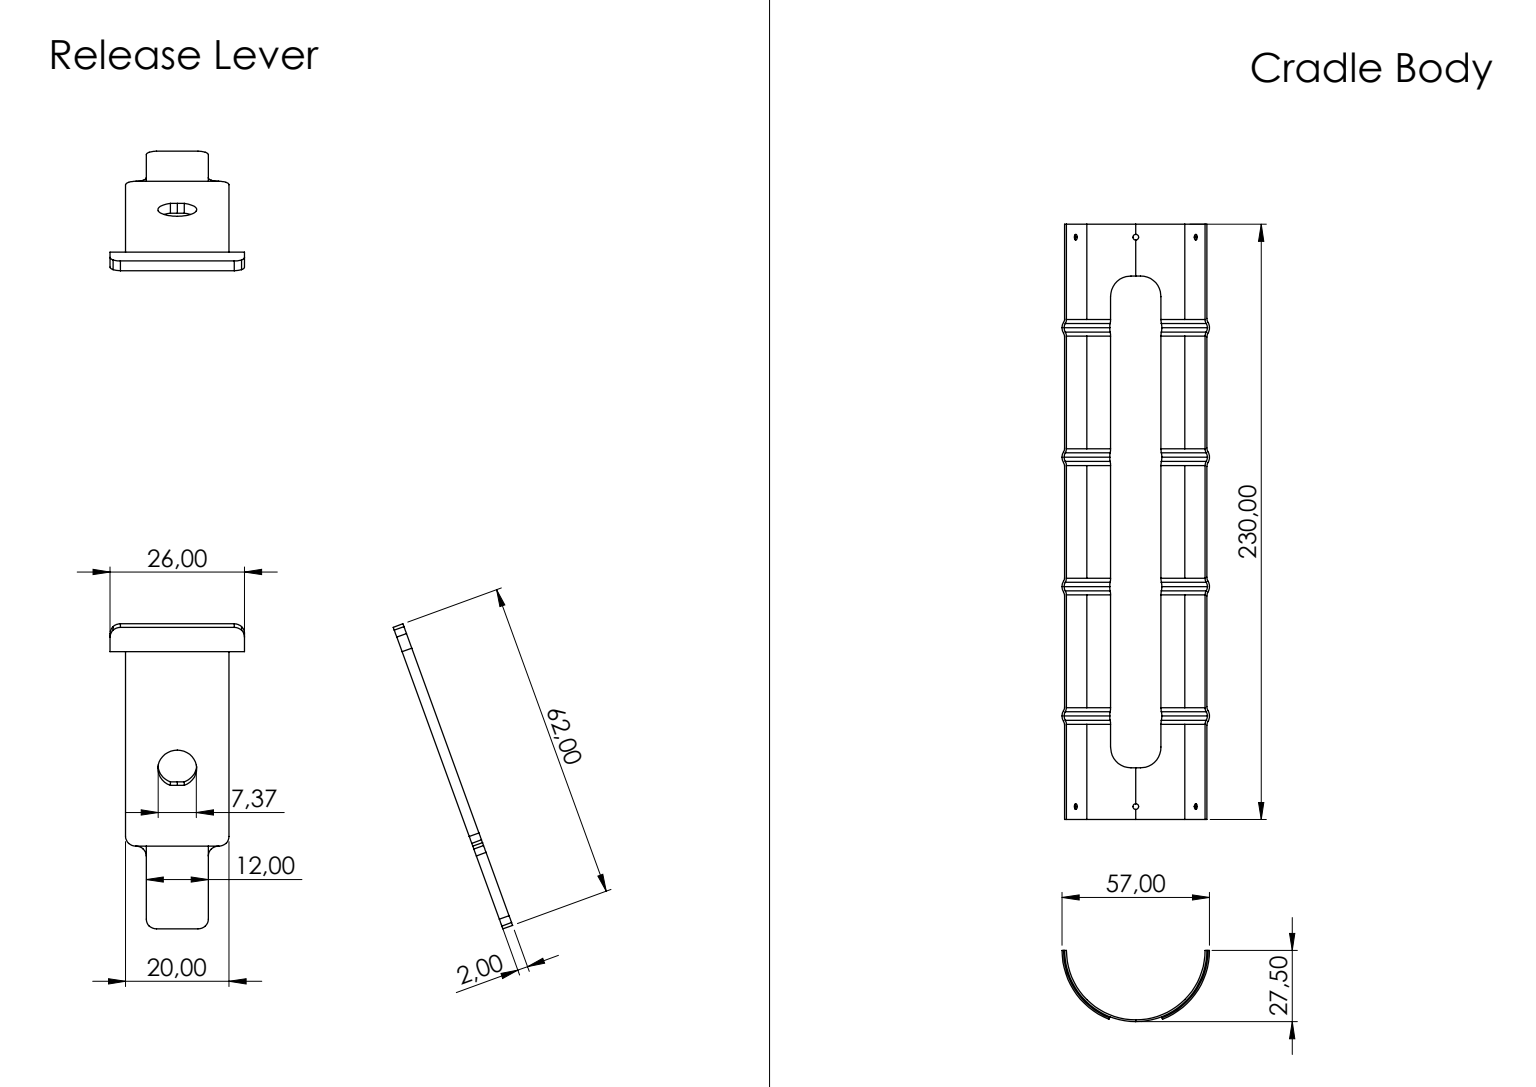
ISO-10303-21;
HEADER;
FILE_DESCRIPTION (('STEP AP214'),
    '1' );
FILE_NAME ('Release Lever.step',
    '2026-10-06T09:00:30',
    ( '' ),
    ( '' ),
    'SwSTEP 2.0',
    'SolidWorks 2020',
    '' );
FILE_SCHEMA (( 'AUTOMOTIVE_DESIGN' ));
ENDSEC;

DATA;
#27=EDGE_CURVE ( 'NONE', #20783, #1709, #15444, .T. ) ;
#39=CARTESIAN_POINT ( 'NONE',  ( 5.746322866173966482, -30.90925660337144265, -80.12837891589188644 ) ) ;
#44=CARTESIAN_POINT ( 'NONE',  ( 1.346291201779999946, -4.118494162357343669, -70.37733883405731206 ) ) ;
#60=CARTESIAN_POINT ( 'NONE',  ( -1.682270644565667439, 2.346032993262427091, -68.02444337080407877 ) ) ;
#66=DIRECTION ( 'NONE',  ( 0.000000000000000000, -0.3420201433259318913, 0.9396926207858126157 ) ) ;
#94=ORIENTED_EDGE ( 'NONE', *, *, #1377, .F. ) ;
#102=CARTESIAN_POINT ( 'NONE',  ( -10.00000000000000000, 21.72305290929948640, -60.97178489257708378 ) ) ;
#116=CARTESIAN_POINT ( 'NONE',  ( -6.000000000000000000, -30.08462078616447499, -79.82823602431849963 ) ) ;
#118=CARTESIAN_POINT ( 'NONE',  ( -8.261799387992772026, -15.86465192213916353, -74.65259062561661096 ) ) ;
#129=AXIS2_PLACEMENT_3D ( 'NONE', #21311, #28843, #21003 ) ;
#132=ORIENTED_EDGE ( 'NONE', *, *, #23382, .F. ) ;
#139=CARTESIAN_POINT ( 'NONE',  ( 0.000000000000000000, 5.495185456771864096, -69.00660115587162124 ) ) ;
#141=CYLINDRICAL_SURFACE ( 'NONE', #31028, 3.749999999999999556 ) ;
#143=CIRCLE ( 'NONE', #28760, 2.000000000000000000 ) ;
#148=CARTESIAN_POINT ( 'NONE',  ( 4.000000000000000000, -31.49740633216590524, -81.40662568294101220 ) ) ;
#151=CARTESIAN_POINT ( 'NONE',  ( 4.000000000000000000, -29.96004123392021157, -79.78289277550334191 ) ) ;
#168=ORIENTED_EDGE ( 'NONE', *, *, #10296, .F. ) ;
#201=DIRECTION ( 'NONE',  ( 0.000000000000000000, 0.3420201433259318913, -0.9396926207858126157 ) ) ;
#218=LINE ( 'NONE', #7132, #8498 ) ;
#267=DIRECTION ( 'NONE',  ( -1.000000000000000000, 0.000000000000000000, 0.000000000000000000 ) ) ;
#348=LINE ( 'NONE', #2999, #25253 ) ;
#359=VERTEX_POINT ( 'NONE', #2030 ) ;
#376=LINE ( 'NONE', #19562, #18555 ) ;
#394=ORIENTED_EDGE ( 'NONE', *, *, #19312, .F. ) ;
#425=DIRECTION ( 'NONE',  ( -1.000000000000000000, 0.000000000000000000, 0.000000000000000000 ) ) ;
#430=CARTESIAN_POINT ( 'NONE',  ( -6.000000000000000000, -29.96004123392021157, -79.78289277550334191 ) ) ;
#446=EDGE_CURVE ( 'NONE', #1677, #8641, #13828, .T. ) ;
#476=AXIS2_PLACEMENT_3D ( 'NONE', #10659, #13016, #25296 ) ;
#506=CARTESIAN_POINT ( 'NONE',  ( 9.229093439197374238, -15.48814874288954613, -74.51555467526300447 ) ) ;
#507=CARTESIAN_POINT ( 'NONE',  ( 5.601646981916513113, -31.11278470850464473, -80.20245708799704687 ) ) ;
#526=FILL_AREA_STYLE_COLOUR ( '', #18851 ) ;
#533=ORIENTED_EDGE ( 'NONE', *, *, #12374, .F. ) ;
#544=APPLICATION_CONTEXT ( 'automotive_design' ) ;
#572=( LENGTH_UNIT ( ) NAMED_UNIT ( * ) SI_UNIT ( .MILLI., .METRE. ) );
#634=ORIENTED_EDGE ( 'NONE', *, *, #28989, .F. ) ;
#639=PRODUCT_CONTEXT ( 'NONE', #19223, 'mechanical' ) ;
#645=CARTESIAN_POINT ( 'NONE',  ( -6.585786437629999490, -15.73107082825028336, -76.73232662853232000 ) ) ;
#653=CARTESIAN_POINT ( 'NONE',  ( 3.686970300939999667, -0.1862064327014488485, -68.94610314789109395 ) ) ;
#665=EDGE_LOOP ( 'NONE', ( #12496, #18069, #19743, #15909 ) ) ;
#670=CARTESIAN_POINT ( 'NONE',  ( 9.947945353310727157, -14.47719179179285476, -74.14759643693901126 ) ) ;
#703=DIRECTION ( 'NONE',  ( -1.000000000000000000, 0.000000000000000000, 0.000000000000000000 ) ) ;
#724=DIRECTION ( 'NONE',  ( 0.000000000000000000, -0.3420201433259318358, 0.9396926207858125046 ) ) ;
#759=AXIS2_PLACEMENT_3D ( 'NONE', #15036, #8234, #5426 ) ;
#767=B_SPLINE_CURVE_WITH_KNOTS ( 'NONE', 3,
 ( #13205, #8639, #22518, #965, #1269, #18235 ),
 .UNSPECIFIED., .F., .F.,
 ( 4, 2, 4 ),
 ( 0.000000000000000000, 0.5000000000000000000, 1.000000000000000000 ),
 .UNSPECIFIED. ) ;
#787=ADVANCED_FACE ( 'NONE', ( #14575 ), #4508, .F. ) ;
#816=CARTESIAN_POINT ( 'NONE',  ( -8.000000000000000000, -17.05999687705277879, -77.21601615383784178 ) ) ;
#826=ORIENTED_EDGE ( 'NONE', *, *, #17759, .F. ) ;
#877=DIRECTION ( 'NONE',  ( -0.000000000000000000, -0.9396926207858126157, -0.3420201433259318913 ) ) ;
#894=ORIENTED_EDGE ( 'NONE', *, *, #4532, .F. ) ;
#933=AXIS2_PLACEMENT_3D ( 'NONE', #27960, #6400, #18514 ) ;
#941=MANIFOLD_SOLID_BREP ( 'PartBody', #9536 ) ;
#949=CARTESIAN_POINT ( 'NONE',  ( 8.000000000050000892, -13.98526668056139144, -73.96855033896248699 ) ) ;
#965=CARTESIAN_POINT ( 'NONE',  ( -9.947945353463017781, -14.47719179108256782, -74.14759643668045896 ) ) ;
#1023=PRESENTATION_STYLE_ASSIGNMENT (( #20206 ) ) ;
#1039=FACE_OUTER_BOUND ( 'NONE', #21921, .T. ) ;
#1080=ORIENTED_EDGE ( 'NONE', *, *, #19351, .T. ) ;
#1104=CARTESIAN_POINT ( 'NONE',  ( -11.50000000000000000, 22.40709319595134730, -62.85117013414870257 ) ) ;
#1176=EDGE_CURVE ( 'NONE', #24619, #15474, #22131, .T. ) ;
#1181=DIRECTION ( 'NONE',  ( 0.9831920802501790124, -0.1715636151751586680, -0.06244404920691486172 ) ) ;
#1199=CARTESIAN_POINT ( 'NONE',  ( 10.00000000000000000, 21.72305290929948640, -60.97178489257708378 ) ) ;
#1210=AXIS2_PLACEMENT_3D ( 'NONE', #8253, #3381, #5296 ) ;
#1247=ORIENTED_EDGE ( 'NONE', *, *, #9957, .T. ) ;
#1248=AXIS2_PLACEMENT_3D ( 'NONE', #26035, #21308, #6364 ) ;
#1269=CARTESIAN_POINT ( 'NONE',  ( -10.00000000005000445, -14.23127763322419703, -74.05809100303530101 ) ) ;
#1274=ORIENTED_EDGE ( 'NONE', *, *, #21907, .T. ) ;
#1281=CARTESIAN_POINT ( 'NONE',  ( 6.000000000000000000, -17.74403716370463968, -75.33663091226621589 ) ) ;
#1284=SURFACE_STYLE_USAGE ( .BOTH. , #7880 ) ;
#1293=CARTESIAN_POINT ( 'NONE',  ( -8.000000000000000000, -17.74403716370463968, -75.33663091226621589 ) ) ;
#1321=CARTESIAN_POINT ( 'NONE',  ( -3.686970300939999667, -0.1862064327014488485, -68.94610314789107974 ) ) ;
#1336=CARTESIAN_POINT ( 'NONE',  ( -4.000000000000000000, -29.27600094726834712, -81.66227801707495360 ) ) ;
#1347=VERTEX_POINT ( 'NONE', #9746 ) ;
#1370=B_SPLINE_CURVE_WITH_KNOTS ( 'NONE', 3,
 ( #653, #3728, #17314, #26919, #19984, #11129, #26759, #24707, #25292, #6250 ),
 .UNSPECIFIED., .F., .F.,
 ( 4, 2, 2, 2, 4 ),
 ( 0.000000000000000000, 0.2500000000000000000, 0.5000000000000000000, 0.7500000000000000000, 1.000000000000000000 ),
 .UNSPECIFIED. ) ;
#1377=EDGE_CURVE ( 'NONE', #21922, #24619, #143, .T. ) ;
#1378=CARTESIAN_POINT ( 'NONE',  ( -8.000000000000000000, -15.86465192213301556, -74.65259062561435144 ) ) ;
#1392=LINE ( 'NONE', #16015, #6709 ) ;
#1399=AXIS2_PLACEMENT_3D ( 'NONE', #949, #20134, #22648 ) ;
#1472=DIRECTION ( 'NONE',  ( 0.000000000000000000, 0.3420201433259318913, -0.9396926207858126157 ) ) ;
#1496=AXIS2_PLACEMENT_3D ( 'NONE', #1293, #13078, #29613 ) ;
#1517=CARTESIAN_POINT ( 'NONE',  ( 1.070547230664766758, 2.553693132251782405, -67.94886126136832161 ) ) ;
#1528=EDGE_CURVE ( 'NONE', #24268, #24784, #17639, .T. ) ;
#1533=CARTESIAN_POINT ( 'NONE',  ( 8.000000000000000000, -15.86465192213301556, -74.65259062561435144 ) ) ;
#1567=EDGE_CURVE ( 'NONE', #13375, #14059, #30931, .T. ) ;
#1573=CARTESIAN_POINT ( 'NONE',  ( 11.00000000000000000, 26.42151601322854759, -59.26168417594741555 ) ) ;
#1597=EDGE_LOOP ( 'NONE', ( #9088, #27743, #23180, #6425 ) ) ;
#1608=VECTOR ( 'NONE', #14619, 1000.000000000000114 ) ;
#1661=CARTESIAN_POINT ( 'NONE',  ( 8.000000000050000892, -13.98526668056139144, -73.96855033896248699 ) ) ;
#1677=VERTEX_POINT ( 'NONE', #1281 ) ;
#1694=DIRECTION ( 'NONE',  ( 0.000000000000000000, 0.3420201433259318358, -0.9396926207858125046 ) ) ;
#1702=ORIENTED_EDGE ( 'NONE', *, *, #26033, .F. ) ;
#1709=VERTEX_POINT ( 'NONE', #28014 ) ;
#1710=CIRCLE ( 'NONE', #5716, 2.000000000000000000 ) ;
#1758=AXIS2_PLACEMENT_3D ( 'NONE', #6175, #1472, #20659 ) ;
#1791=LINE ( 'NONE', #25394, #9769 ) ;
#1855=LINE ( 'NONE', #16324, #16326 ) ;
#1890=LINE ( 'NONE', #6760, #17257 ) ;
#1892=EDGE_CURVE ( 'NONE', #3795, #15436, #7619, .T. ) ;
#1894=CARTESIAN_POINT ( 'NONE',  ( -3.629744515141296368, -1.804033921010813835, -69.53494419781382874 ) ) ;
#1895=ORIENTED_EDGE ( 'NONE', *, *, #2972, .T. ) ;
#1912=AXIS2_PLACEMENT_3D ( 'NONE', #21616, #66, #9646 ) ;
#1918=PLANE ( 'NONE',  #23555 ) ;
#1930=CARTESIAN_POINT ( 'NONE',  ( -6.000000000000000000, -23.85203919881242385, -77.55976184388477179 ) ) ;
#1939=ORIENTED_EDGE ( 'NONE', *, *, #28404, .T. ) ;
#1980=CARTESIAN_POINT ( 'NONE',  ( 0.000000000000000000, 27.10555629988041204, -61.14106941751904856 ) ) ;
#1986=ADVANCED_FACE ( 'NONE', ( #30114, #6190 ), #13906, .F. ) ;
#1999=LINE ( 'NONE', #29299, #4426 ) ;
#2027=ORIENTED_EDGE ( 'NONE', *, *, #20844, .F. ) ;
#2030=CARTESIAN_POINT ( 'NONE',  ( -10.00000000000000000, -13.98526668056139144, -73.96855033896248699 ) ) ;
#2106=DIRECTION ( 'NONE',  ( 0.000000000000000000, -0.3420201433259318913, 0.9396926207858126157 ) ) ;
#2111=VERTEX_POINT ( 'NONE', #9019 ) ;
#2145=ORIENTED_EDGE ( 'NONE', *, *, #29497, .T. ) ;
#2148=DIRECTION ( 'NONE',  ( 0.000000000000000000, -0.3420201433259318358, 0.9396926207858125046 ) ) ;
#2167=CARTESIAN_POINT ( 'NONE',  ( 12.41421356240000051, 26.55509710711128335, -61.34142017886538412 ) ) ;
#2201=LINE ( 'NONE', #4866, #16643 ) ;
#2209=CARTESIAN_POINT ( 'NONE',  ( -1.750888960315145848, -3.972249423281244862, -70.32411010211554014 ) ) ;
#2211=CIRCLE ( 'NONE', #10247, 3.750000000000000000 ) ;
#2254=DIRECTION ( 'NONE',  ( 0.000000000000000000, 0.9396926207858125046, 0.3420201433259318358 ) ) ;
#2256=EDGE_LOOP ( 'NONE', ( #634, #29786, #11374, #18353 ) ) ;
#2258=VERTEX_POINT ( 'NONE', #26478 ) ;
#2291=FACE_OUTER_BOUND ( 'NONE', #5378, .T. ) ;
#2296=( GEOMETRIC_REPRESENTATION_CONTEXT ( 3 ) GLOBAL_UNCERTAINTY_ASSIGNED_CONTEXT ( ( #10001 ) ) GLOBAL_UNIT_ASSIGNED_CONTEXT ( ( #15439, #3164, #8338 ) ) REPRESENTATION_CONTEXT ( 'NONE', 'WORKASPACE' ) );
#2356=LINE ( 'NONE', #16655, #3079 ) ;
#2365=CARTESIAN_POINT ( 'NONE',  ( 5.999999999999997335, -17.49802621104079137, -75.24709024819303238 ) ) ;
#2368=ORIENTED_EDGE ( 'NONE', *, *, #11363, .T. ) ;
#2392=CARTESIAN_POINT ( 'NONE',  ( 8.261799387612766665, -15.86465192213917064, -74.65259062561659675 ) ) ;
#2433=DIRECTION ( 'NONE',  ( -1.000000000000000000, 0.000000000000000000, 0.000000000000000000 ) ) ;
#2440=DIRECTION ( 'NONE',  ( 0.000000000000000000, 0.3420201433259318913, -0.9396926207858126157 ) ) ;
#2442=VECTOR ( 'NONE', #2526, 1000.000000000000114 ) ;
#2468=CARTESIAN_POINT ( 'NONE',  ( -13.00000000000000000, 23.81663212713006672, -62.33813991915980779 ) ) ;
#2526=DIRECTION ( 'NONE',  ( 0.000000000000000000, 0.3420201433259318358, -0.9396926207858125046 ) ) ;
#2539=DIRECTION ( 'NONE',  ( 0.000000000000000000, -0.9396926207858125046, -0.3420201433259318358 ) ) ;
#2540=VECTOR ( 'NONE', #17749, 1000.000000000000114 ) ;
#2569=DIRECTION ( 'NONE',  ( 0.000000000000000000, 0.3420201433259318913, -0.9396926207858126157 ) ) ;
#2573=AXIS2_PLACEMENT_3D ( 'NONE', #24001, #2440, #18795 ) ;
#2616=CARTESIAN_POINT ( 'NONE',  ( 1.243449787579999883E-14, -31.15538618883996946, -82.34631830372681804 ) ) ;
#2627=CARTESIAN_POINT ( 'NONE',  ( 0.000000000000000000, 0.000000000000000000, 0.000000000000000000 ) ) ;
#2633=ORIENTED_EDGE ( 'NONE', *, *, #7472, .F. ) ;
#2672=VERTEX_POINT ( 'NONE', #14752 ) ;
#2691=CARTESIAN_POINT ( 'NONE',  ( 12.74757277707238856, 25.48862485010116075, -59.60122879113606587 ) ) ;
#2695=EDGE_CURVE ( 'NONE', #22118, #18765, #4850, .T. ) ;
#2708=CARTESIAN_POINT ( 'NONE',  ( 9.747572776401462136, -14.93176076027399901, -74.31304601088737627 ) ) ;
#2762=CARTESIAN_POINT ( 'NONE',  ( -11.00000000000000000, 25.22617105830878614, -61.82510970417090590 ) ) ;
#2772=CARTESIAN_POINT ( 'NONE',  ( -0.6731456008920000400, -3.434453875705480108, -72.25672407562892374 ) ) ;
#2813=CYLINDRICAL_SURFACE ( 'NONE', #24284, 2.000000000000003553 ) ;
#2814=LINE ( 'NONE', #22167, #18267 ) ;
#2817=ADVANCED_FACE ( 'NONE', ( #24932 ), #22423, .F. ) ;
#2827=ORIENTED_EDGE ( 'NONE', *, *, #2972, .F. ) ;
#2869=ORIENTED_EDGE ( 'NONE', *, *, #5232, .T. ) ;
#2891=LINE ( 'NONE', #17205, #10294 ) ;
#2917=CARTESIAN_POINT ( 'NONE',  ( -11.50000000000000000, 22.40709319595134730, -62.85117013414870257 ) ) ;
#2920=DIRECTION ( 'NONE',  ( 1.000000000000000000, -0.000000000000000000, 0.000000000000000000 ) ) ;
#2942=VECTOR ( 'NONE', #8951, 1000.000000000000114 ) ;
#2972=EDGE_CURVE ( 'NONE', #28085, #1347, #19245, .T. ) ;
#2975=EDGE_LOOP ( 'NONE', ( #13463, #826, #26860, #5305, #15473, #13542, #20696, #23812, #24583, #29901 ) ) ;
#2999=CARTESIAN_POINT ( 'NONE',  ( -13.00000000000000000, 22.06507305262541863, -61.91147751336289673 ) ) ;
#3020=EDGE_CURVE ( 'NONE', #31086, #17565, #15659, .T. ) ;
#3067=FACE_OUTER_BOUND ( 'NONE', #13010, .T. ) ;
#3075=EDGE_CURVE ( 'NONE', #359, #15474, #7131, .T. ) ;
#3079=VECTOR ( 'NONE', #21701, 1000.000000000000000 ) ;
#3103=AXIS2_PLACEMENT_3D ( 'NONE', #24128, #2106, #14381 ) ;
#3121=VERTEX_POINT ( 'NONE', #9644 ) ;
#3124=ORIENTED_EDGE ( 'NONE', *, *, #10955, .T. ) ;
#3156=CARTESIAN_POINT ( 'NONE',  ( -5.226724280842381276, -31.46509748598739975, -80.33068845215250064 ) ) ;
#3162=ORIENTED_EDGE ( 'NONE', *, *, #7689, .F. ) ;
#3164=( NAMED_UNIT ( * ) PLANE_ANGLE_UNIT ( ) SI_UNIT ( $, .RADIAN. ) );
#3201=EDGE_CURVE ( 'NONE', #24684, #1347, #376, .T. ) ;
#3202=ORIENTED_EDGE ( 'NONE', *, *, #23759, .F. ) ;
#3277=DIRECTION ( 'NONE',  ( 0.000000000000000000, -0.3420201433259318913, 0.9396926207858126157 ) ) ;
#3280=ORIENTED_EDGE ( 'NONE', *, *, #21019, .F. ) ;
#3293=LINE ( 'NONE', #24402, #27778 ) ;
#3364=DIRECTION ( 'NONE',  ( 0.000000000000000000, -0.9396926207858125046, -0.3420201433259318358 ) ) ;
#3381=DIRECTION ( 'NONE',  ( 0.000000000000000000, 0.3420201433259318913, -0.9396926207858126157 ) ) ;
#3396=AXIS2_PLACEMENT_3D ( 'NONE', #10919, #6031, #8542 ) ;
#3414=DIRECTION ( 'NONE',  ( 0.000000000000000000, 0.3420201433259318913, -0.9396926207858126157 ) ) ;
#3449=DIRECTION ( 'NONE',  ( 0.000000000000000000, 0.3420201433259318913, -0.9396926207858126157 ) ) ;
#3456=CARTESIAN_POINT ( 'NONE',  ( 9.414213562409999625, -15.31419272936388687, -74.45223986426802298 ) ) ;
#3462=CARTESIAN_POINT ( 'NONE',  ( -4.000000000000000000, -31.83942647549183746, -80.46693306215520636 ) ) ;
#3463=ORIENTED_EDGE ( 'NONE', *, *, #18343, .T. ) ;
#3464=CARTESIAN_POINT ( 'NONE',  ( -11.00000000000000000, 27.10555629988041204, -61.14106941751904856 ) ) ;
#3466=ORIENTED_EDGE ( 'NONE', *, *, #9897, .T. ) ;
#3472=ORIENTED_EDGE ( 'NONE', *, *, #15387, .T. ) ;
#3481=EDGE_CURVE ( 'NONE', #2258, #24119, #10233, .T. ) ;
#3495=B_SPLINE_CURVE_WITH_KNOTS ( 'NONE', 3,
 ( #19220, #21591, #2691, #7107, #26304, #28969 ),
 .UNSPECIFIED., .F., .F.,
 ( 4, 2, 4 ),
 ( 0.000000000000000000, 0.5000000000000000000, 1.000000000000000000 ),
 .UNSPECIFIED. ) ;
#3521=ORIENTED_EDGE ( 'NONE', *, *, #29385, .F. ) ;
#3570=DIRECTION ( 'NONE',  ( 0.7071067811865467956, 0.6644630243886068266, 0.2418447626481644297 ) ) ;
#3628=VECTOR ( 'NONE', #19062, 1000.000000000000114 ) ;
#3630=CARTESIAN_POINT ( 'NONE',  ( -3.015466128627334985, 1.304460199876133819, -68.40354486441854931 ) ) ;
#3636=CARTESIAN_POINT ( 'NONE',  ( -12.41421356240000051, 25.87105682045942245, -59.46203493729375822 ) ) ;
#3649=CARTESIAN_POINT ( 'NONE',  ( 4.440892098500000496E-16, -0.1455297029551360921, -71.05965357398815740 ) ) ;
#3674=CARTESIAN_POINT ( 'NONE',  ( 6.000000000000000000, -23.16799891216055940, -79.43914708545641190 ) ) ;
#3689=FACE_OUTER_BOUND ( 'NONE', #23976, .T. ) ;
#3706=DIRECTION ( 'NONE',  ( -1.000000000000000000, 0.000000000000000000, 0.000000000000000000 ) ) ;
#3721=AXIS2_PLACEMENT_3D ( 'NONE', #2917, #877, #425 ) ;
#3726=LINE ( 'NONE', #30323, #10479 ) ;
#3728=CARTESIAN_POINT ( 'NONE',  ( 3.766879923516746942, -0.5905747970024824989, -69.09328119617570962 ) ) ;
#3744=AXIS2_PLACEMENT_3D ( 'NONE', #31113, #5131, #14744 ) ;
#3783=VECTOR ( 'NONE', #2539, 1000.000000000000114 ) ;
#3795=VERTEX_POINT ( 'NONE', #19012 ) ;
#3796=( NAMED_UNIT ( * ) PLANE_ANGLE_UNIT ( ) SI_UNIT ( $, .RADIAN. ) );
#3810=EDGE_CURVE ( 'NONE', #359, #7467, #16800, .T. ) ;
#3866=CARTESIAN_POINT ( 'NONE',  ( 3.454291557259786316, 0.6014336072404916633, -68.65942561803572630 ) ) ;
#3913=VECTOR ( 'NONE', #4734, 1000.000000000000114 ) ;
#3924=CARTESIAN_POINT ( 'NONE',  ( 8.000000000000000000, -15.86465192213301556, -74.65259062561435144 ) ) ;
#3961=CARTESIAN_POINT ( 'NONE',  ( -12.22909343913021551, 26.04501283399531530, -59.39872012629501086 ) ) ;
#4004=VECTOR ( 'NONE', #18311, 1000.000000000000000 ) ;
#4017=ORIENTED_EDGE ( 'NONE', *, *, #7464, .F. ) ;
#4024=CARTESIAN_POINT ( 'NONE',  ( 0.8593139071816520147, 2.606839092805549818, -67.92951771365525815 ) ) ;
#4032=ORIENTED_EDGE ( 'NONE', *, *, #27, .T. ) ;
#4062=ORIENTED_EDGE ( 'NONE', *, *, #14447, .F. ) ;
#4102=EDGE_LOOP ( 'NONE', ( #533, #28019, #19197, #15165, #11526, #3521, #18884, #25233, #20427, #3466 ) ) ;
#4198=CIRCLE ( 'NONE', #26331, 3.750000000000000000 ) ;
#4356=EDGE_LOOP ( 'NONE', ( #12880, #9635, #28055, #16249 ) ) ;
#4360=CARTESIAN_POINT ( 'NONE',  ( -1.346291201779999946, -4.118494162357343669, -70.37733883405731206 ) ) ;
#4383=LINE ( 'NONE', #11156, #20990 ) ;
#4418=ORIENTED_EDGE ( 'NONE', *, *, #30801, .F. ) ;
#4426=VECTOR ( 'NONE', #26640, 1000.000000000000114 ) ;
#4440=DIRECTION ( 'NONE',  ( 0.000000000000000000, 0.3420201433259318358, -0.9396926207858125046 ) ) ;
#4503=AXIS2_PLACEMENT_3D ( 'NONE', #17531, #27139, #21653 ) ;
#4508=PLANE ( 'NONE',  #25624 ) ;
#4532=EDGE_CURVE ( 'NONE', #9238, #25602, #14330, .T. ) ;
#4538=DIRECTION ( 'NONE',  ( -1.000000000000000000, 0.000000000000000000, 0.000000000000000000 ) ) ;
#4574=LINE ( 'NONE', #11966, #3913 ) ;
#4587=EDGE_CURVE ( 'NONE', #8607, #4930, #20356, .T. ) ;
#4687=EDGE_LOOP ( 'NONE', ( #26398, #94, #9751, #13440 ) ) ;
#4709=ADVANCED_FACE ( 'NONE', ( #11706 ), #28225, .T. ) ;
#4713=VECTOR ( 'NONE', #19034, 1000.000000000000114 ) ;
#4734=DIRECTION ( 'NONE',  ( 0.000000000000000000, 0.3420201433259318358, -0.9396926207858125046 ) ) ;
#4753=CARTESIAN_POINT ( 'NONE',  ( 9.007237960087341122, -15.62744792347586476, -74.56625543065413808 ) ) ;
#4766=CARTESIAN_POINT ( 'NONE',  ( -11.00000000000000000, 25.22617105830878614, -61.82510970417090590 ) ) ;
#4836=ADVANCED_FACE ( 'NONE', ( #29152 ), #14226, .F. ) ;
#4848=B_SPLINE_CURVE_WITH_KNOTS ( 'NONE', 3,
 ( #9368, #29150, #10122, #7597, #11739, #17190 ),
 .UNSPECIFIED., .F., .F.,
 ( 4, 2, 4 ),
 ( 0.000000000000000000, 0.5000000000000000000, 1.000000000000000000 ),
 .UNSPECIFIED. ) ;
#4850=LINE ( 'NONE', #10033, #10148 ) ;
#4853=DIRECTION ( 'NONE',  ( 0.000000000000000000, 0.3420201433259318913, -0.9396926207858126157 ) ) ;
#4866=CARTESIAN_POINT ( 'NONE',  ( -6.339027081030000540E-10, -3.776474019031412777, -71.31703145484311790 ) ) ;
#4870=CARTESIAN_POINT ( 'NONE',  ( 13.00000000000000000, 22.40709319595134730, -62.85117013414870257 ) ) ;
#4884=CARTESIAN_POINT ( 'NONE',  ( 6.000000000000000000, -17.74403716370463968, -75.33663091226621589 ) ) ;
#4886=ORIENTED_EDGE ( 'NONE', *, *, #14233, .F. ) ;
#4930=VERTEX_POINT ( 'NONE', #6005 ) ;
#4972=PLANE ( 'NONE',  #3721 ) ;
#4976=CARTESIAN_POINT ( 'NONE',  ( -5.936576268373215726, -30.44659052782209585, -79.95998223598701315 ) ) ;
#4990=FACE_OUTER_BOUND ( 'NONE', #14209, .T. ) ;
#5015=DIRECTION ( 'NONE',  ( -1.000000000000000000, 0.000000000000000000, 0.000000000000000000 ) ) ;
#5018=DIRECTION ( 'NONE',  ( 0.000000000000000000, 0.3420201433259318913, -0.9396926207858126157 ) ) ;
#5064=ORIENTED_EDGE ( 'NONE', *, *, #15160, .F. ) ;
#5131=DIRECTION ( 'NONE',  ( 0.000000000000000000, 0.3420201433259318913, -0.9396926207858126157 ) ) ;
#5192=ADVANCED_FACE ( 'NONE', ( #30409 ), #25690, .T. ) ;
#5200=LINE ( 'NONE', #30611, #10649 ) ;
#5232=EDGE_CURVE ( 'NONE', #2258, #2672, #26150, .T. ) ;
#5276=FILL_AREA_STYLE_COLOUR ( '', #6386 ) ;
#5288=LINE ( 'NONE', #2772, #10747 ) ;
#5295=STYLED_ITEM ( 'NONE', ( #18094 ), #9916 ) ;
#5296=DIRECTION ( 'NONE',  ( 0.000000000000000000, 0.9396926207858125046, 0.3420201433259318358 ) ) ;
#5305=ORIENTED_EDGE ( 'NONE', *, *, #25713, .T. ) ;
#5308=PRODUCT_DEFINITION_FORMATION_WITH_SPECIFIED_SOURCE ( 'ANY', '', #28241, .NOT_KNOWN. ) ;
#5345=CARTESIAN_POINT ( 'NONE',  ( -10.00000000000000000, 4.552933401020911042, -69.34955285734142194 ) ) ;
#5353=EDGE_LOOP ( 'NONE', ( #14979, #20824, #16001, #18891 ) ) ;
#5356=CARTESIAN_POINT ( 'NONE',  ( -7.867425209648341244, -15.86465192213301911, -74.65259062561435144 ) ) ;
#5368=VECTOR ( 'NONE', #12353, 1000.000000000000114 ) ;
#5377=EDGE_CURVE ( 'NONE', #9001, #24684, #1370, .T. ) ;
#5378=EDGE_LOOP ( 'NONE', ( #11345, #18822, #7457, #14477 ) ) ;
#5387=EDGE_CURVE ( 'NONE', #16796, #5989, #6660, .T. ) ;
#5426=DIRECTION ( 'NONE',  ( -1.000000000000000000, 0.000000000000000000, 0.000000000000000000 ) ) ;
#5451=VECTOR ( 'NONE', #24263, 1000.000000000000114 ) ;
#5532=CARTESIAN_POINT ( 'NONE',  ( -3.607824829760114760, 0.2143012804528021953, -68.80033026170877974 ) ) ;
#5571=AXIS2_PLACEMENT_3D ( 'NONE', #9859, #7495, #17089 ) ;
#5573=CYLINDRICAL_SURFACE ( 'NONE', #15534, 2.000000000000002665 ) ;
#5589=CARTESIAN_POINT ( 'NONE',  ( -9.229093440751908517, -15.48814874182538226, -74.51555467487568762 ) ) ;
#5654=ADVANCED_FACE ( 'NONE', ( #3689 ), #17994, .F. ) ;
#5705=ORIENTED_EDGE ( 'NONE', *, *, #1176, .F. ) ;
#5716=AXIS2_PLACEMENT_3D ( 'NONE', #816, #10406, #14977 ) ;
#5731=CARTESIAN_POINT ( 'NONE',  ( 6.000000000000000000, -16.12030425626696939, -76.87399601051191667 ) ) ;
#5740=VECTOR ( 'NONE', #13256, 1000.000000000000000 ) ;
#5747=ORIENTED_EDGE ( 'NONE', *, *, #19483, .T. ) ;
#5762=ORIENTED_EDGE ( 'NONE', *, *, #16574, .T. ) ;
#5788=CARTESIAN_POINT ( 'NONE',  ( 13.00000000000000000, 23.81663212713006672, -62.33813991915980779 ) ) ;
#5886=FACE_OUTER_BOUND ( 'NONE', #2256, .T. ) ;
#5900=AXIS2_PLACEMENT_3D ( 'NONE', #14288, #24651, #14748 ) ;
#5929=FACE_OUTER_BOUND ( 'NONE', #24195, .T. ) ;
#5943=AXIS2_PLACEMENT_3D ( 'NONE', #15885, #13838, #6747 ) ;
#5989=VERTEX_POINT ( 'NONE', #22399 ) ;
#6005=CARTESIAN_POINT ( 'NONE',  ( -5.414213562369999622, -30.60492699607083722, -82.14596754238048959 ) ) ;
#6007=DIRECTION ( 'NONE',  ( 0.000000000000000000, 0.3420201433259318358, -0.9396926207858125046 ) ) ;
#6028=DIRECTION ( 'NONE',  ( 0.000000000000000000, 0.3420201433259318913, -0.9396926207858126157 ) ) ;
#6031=DIRECTION ( 'NONE',  ( 0.000000000000000000, -0.3420201433259318913, 0.9396926207858126157 ) ) ;
#6035=DIRECTION ( 'NONE',  ( 0.000000000000000000, -0.9396926207858125046, -0.3420201433259318358 ) ) ;
#6108=VECTOR ( 'NONE', #9491, 1000.000000000000114 ) ;
#6118=CARTESIAN_POINT ( 'NONE',  ( 12.41421356240000051, 25.87105682045942245, -59.46203493729375822 ) ) ;
#6131=CARTESIAN_POINT ( 'NONE',  ( -11.00000000000000000, 27.10555629988041204, -61.14106941751904856 ) ) ;
#6133=ORIENTED_EDGE ( 'NONE', *, *, #1528, .T. ) ;
#6175=CARTESIAN_POINT ( 'NONE',  ( 0.000000000000000000, 4.811145170119999648, -67.12721591429999535 ) ) ;
#6190=FACE_OUTER_BOUND ( 'NONE', #19033, .T. ) ;
#6211=DIRECTION ( 'NONE',  ( 0.000000000000000000, 0.3420201433259318913, -0.9396926207858126157 ) ) ;
#6216=VECTOR ( 'NONE', #9116, 1000.000000000000114 ) ;
#6250=CARTESIAN_POINT ( 'NONE',  ( 1.346291201779999946, -4.118494162357343669, -70.37733883405731206 ) ) ;
#6273=ORIENTED_EDGE ( 'NONE', *, *, #12374, .T. ) ;
#6302=CARTESIAN_POINT ( 'NONE',  ( -1.346291201779999946, -4.118494162357343669, -70.37733883405731206 ) ) ;
#6327=LINE ( 'NONE', #20645, #14528 ) ;
#6337=CARTESIAN_POINT ( 'NONE',  ( 2.664535259099999805E-15, 2.694277338339796213, -67.89769279494430521 ) ) ;
#6364=DIRECTION ( 'NONE',  ( 0.000000000000000000, 0.9396926207858125046, 0.3420201433259318358 ) ) ;
#6386=COLOUR_RGB ( '', 0.66274510, 0.83137255, 0.94901961) ;
#6400=DIRECTION ( 'NONE',  ( 0.000000000000000000, 0.3420201433259318913, -0.9396926207858126157 ) ) ;
#6425=ORIENTED_EDGE ( 'NONE', *, *, #29890, .T. ) ;
#6428=ORIENTED_EDGE ( 'NONE', *, *, #23291, .T. ) ;
#6452=B_SPLINE_CURVE_WITH_KNOTS ( 'NONE', 3,
 ( #22055, #506, #4753, #22199, #2392, #10090 ),
 .UNSPECIFIED., .F., .F.,
 ( 4, 2, 4 ),
 ( 0.000000000000000000, 0.5000000000000000000, 1.000000000000000000 ),
 .UNSPECIFIED. ) ;
#6473=VERTEX_POINT ( 'NONE', #16713 ) ;
#6484=CARTESIAN_POINT ( 'NONE',  ( 0.000000000000000000, 4.811145170119999648, -67.12721591429999535 ) ) ;
#6529=CYLINDRICAL_SURFACE ( 'NONE', #12771, 2.000000000000000000 ) ;
#6563=EDGE_CURVE ( 'NONE', #22118, #27093, #29447, .T. ) ;
#6585=AXIS2_PLACEMENT_3D ( 'NONE', #9296, #7252, #11663 ) ;
#6592=PLANE ( 'NONE',  #5943 ) ;
#6606=CARTESIAN_POINT ( 'NONE',  ( 5.228182028002445136, -31.46370949612416723, -80.33018326515686169 ) ) ;
#6650=CIRCLE ( 'NONE', #15180, 2.000000000000000000 ) ;
#6659=CARTESIAN_POINT ( 'NONE',  ( 6.585786437629999490, -16.41511111490214603, -74.85294138696069410 ) ) ;
#6660=B_SPLINE_CURVE_WITH_KNOTS ( 'NONE', 3,
 ( #1378, #5356, #27068, #14961, #13327, #10088, #27639, #12588 ),
 .UNSPECIFIED., .F., .F.,
 ( 4, 2, 2, 4 ),
 ( 0.000000000000000000, 0.2499999999999985567, 0.4999999999999971134, 1.000000000000000000 ),
 .UNSPECIFIED. ) ;
#6709=VECTOR ( 'NONE', #30806, 1000.000000000000114 ) ;
#6741=CARTESIAN_POINT ( 'NONE',  ( -10.00000000000000000, 3.868893114322062843, -67.47016761578689170 ) ) ;
#6742=CARTESIAN_POINT ( 'NONE',  ( -9.414213562409999625, -15.31419272936388687, -74.45223986426802298 ) ) ;
#6747=DIRECTION ( 'NONE',  ( -1.000000000000000000, 0.000000000000000000, 0.000000000000000000 ) ) ;
#6757=AXIS2_PLACEMENT_3D ( 'NONE', #4766, #201, #19393 ) ;
#6760=CARTESIAN_POINT ( 'NONE',  ( 11.50000000000000000, 21.72305290929948640, -60.97178489257708378 ) ) ;
#6767=DIRECTION ( 'NONE',  ( 0.000000000000000000, 0.3420201433259318913, -0.9396926207858126157 ) ) ;
#6792=MECHANICAL_DESIGN_GEOMETRIC_PRESENTATION_REPRESENTATION('',(#5295),#16853);
#6812=ORIENTED_EDGE ( 'NONE', *, *, #23979, .F. ) ;
#6837=DIRECTION ( 'NONE',  ( -1.000000000000000000, 0.000000000000000000, 0.000000000000000000 ) ) ;
#6838=EDGE_LOOP ( 'NONE', ( #27624, #2869, #28249, #29286 ) ) ;
#6915=AXIS2_PLACEMENT_3D ( 'NONE', #7197, #12381, #21989 ) ;
#6935=SHAPE_REPRESENTATION ( 'Release Lever', ( #17722 ), #2296 ) ;
#6984=ORIENTED_EDGE ( 'NONE', *, *, #19106, .T. ) ;
#7073=EDGE_CURVE ( 'NONE', #15474, #20783, #12731, .T. ) ;
#7075=VERTEX_POINT ( 'NONE', #18183 ) ;
#7100=ORIENTED_EDGE ( 'NONE', *, *, #23883, .F. ) ;
#7107=CARTESIAN_POINT ( 'NONE',  ( 12.94794535341399389, 25.03405588217355415, -59.76667836488295649 ) ) ;
#7109=CIRCLE ( 'NONE', #7596, 2.000000000000000000 ) ;
#7130=VECTOR ( 'NONE', #28397, 1000.000000000000114 ) ;
#7131=LINE ( 'NONE', #14534, #6108 ) ;
#7132=CARTESIAN_POINT ( 'NONE',  ( -11.50000000000000000, 21.72305290929948640, -60.97178489257708378 ) ) ;
#7188=CARTESIAN_POINT ( 'NONE',  ( -6.253676594953650358, -16.79482187635032986, -74.99114480175852293 ) ) ;
#7197=CARTESIAN_POINT ( 'NONE',  ( -13.00000000000000000, 23.81663212713006672, -62.33813991915980779 ) ) ;
#7252=DIRECTION ( 'NONE',  ( 0.000000000000000000, -0.3420201433259318913, 0.9396926207858126157 ) ) ;
#7265=CARTESIAN_POINT ( 'NONE',  ( 5.949264573234793296, -30.44932768689938740, -79.96097848041759448 ) ) ;
#7286=CARTESIAN_POINT ( 'NONE',  ( -2.730738507911396606, 1.619674855095874610, -68.28881611251394190 ) ) ;
#7326=ADVANCED_FACE ( 'NONE', ( #24312 ), #5573, .T. ) ;
#7328=CARTESIAN_POINT ( 'NONE',  ( 7.000000000000000000, -15.18061163548115466, -76.53197586718597734 ) ) ;
#7360=ORIENTED_EDGE ( 'NONE', *, *, #25956, .T. ) ;
#7398=CARTESIAN_POINT ( 'NONE',  ( 10.00000000000000000, 3.868893114322062843, -67.47016761578689170 ) ) ;
#7416=VECTOR ( 'NONE', #14110, 1000.000000000000114 ) ;
#7426=ORIENTED_EDGE ( 'NONE', *, *, #29497, .F. ) ;
#7431=EDGE_LOOP ( 'NONE', ( #20709, #19090, #6812, #15584 ) ) ;
#7451=CARTESIAN_POINT ( 'NONE',  ( 0.000000000000000000, -3.434453875705480108, -72.25672407562892374 ) ) ;
#7457=ORIENTED_EDGE ( 'NONE', *, *, #9897, .F. ) ;
#7464=EDGE_CURVE ( 'NONE', #26031, #29777, #21083, .T. ) ;
#7467=VERTEX_POINT ( 'NONE', #102 ) ;
#7472=EDGE_CURVE ( 'NONE', #10219, #19754, #19286, .T. ) ;
#7493=CARTESIAN_POINT ( 'NONE',  ( -8.523495769106718356, -15.81573655472489470, -74.63478688787961346 ) ) ;
#7495=DIRECTION ( 'NONE',  ( -1.000000000000000000, -0.000000000000000000, 0.000000000000000000 ) ) ;
#7503=ORIENTED_EDGE ( 'NONE', *, *, #12189, .T. ) ;
#7544=VERTEX_POINT ( 'NONE', #27439 ) ;
#7592=DIRECTION ( 'NONE',  ( 0.000000000000000000, 0.3420201433259318358, -0.9396926207858125046 ) ) ;
#7596=AXIS2_PLACEMENT_3D ( 'NONE', #29083, #22014, #5015 ) ;
#7597=CARTESIAN_POINT ( 'NONE',  ( -12.74757277634464003, 25.48862485138152678, -59.60122879067003510 ) ) ;
#7619=LINE ( 'NONE', #17828, #9955 ) ;
#7638=CARTESIAN_POINT ( 'NONE',  ( -5.897866114205988275, -30.56559748946277466, -80.00329722769471630 ) ) ;
#7671=FACE_OUTER_BOUND ( 'NONE', #28980, .T. ) ;
#7689=EDGE_CURVE ( 'NONE', #12087, #7467, #218, .T. ) ;
#7699=FACE_OUTER_BOUND ( 'NONE', #8652, .T. ) ;
#7733=VECTOR ( 'NONE', #22597, 1000.000000000000000 ) ;
#7743=CYLINDRICAL_SURFACE ( 'NONE', #24037, 2.000000000000003553 ) ;
#7769=ORIENTED_EDGE ( 'NONE', *, *, #24497, .T. ) ;
#7797=ADVANCED_FACE ( 'NONE', ( #22686 ), #29457, .F. ) ;
#7827=CARTESIAN_POINT ( 'NONE',  ( -6.000000000000000000, -15.86465192213301556, -74.65259062561435144 ) ) ;
#7880=SURFACE_SIDE_STYLE ('',( #29290 ) ) ;
#7940=VECTOR ( 'NONE', #23938, 1000.000000000000000 ) ;
#7947=DIRECTION ( 'NONE',  ( 0.000000000000000000, 0.3420201433259318913, -0.9396926207858126157 ) ) ;
#7975=AXIS2_PLACEMENT_3D ( 'NONE', #18820, #16000, #13796 ) ;
#8004=CYLINDRICAL_SURFACE ( 'NONE', #1399, 1.999999999999999334 ) ;
#8103=VERTEX_POINT ( 'NONE', #6742 ) ;
#8147=VERTEX_POINT ( 'NONE', #28922 ) ;
#8201=LINE ( 'NONE', #24749, #22074 ) ;
#8215=AXIS2_PLACEMENT_3D ( 'NONE', #28705, #28084, #6837 ) ;
#8230=( NAMED_UNIT ( * ) PLANE_ANGLE_UNIT ( ) SI_UNIT ( $, .RADIAN. ) );
#8231=ADVANCED_FACE ( 'NONE', ( #26563 ), #141, .F. ) ;
#8234=DIRECTION ( 'NONE',  ( 0.000000000000000000, -0.3420201433259318913, 0.9396926207858126157 ) ) ;
#8249=CARTESIAN_POINT ( 'NONE',  ( 11.00000000000000000, 25.22617105830878614, -61.82510970417090590 ) ) ;
#8253=CARTESIAN_POINT ( 'NONE',  ( 0.000000000000000000, 5.495185456771864096, -69.00660115587162124 ) ) ;
#8276=CARTESIAN_POINT ( 'NONE',  ( -6.000000000000000000, -29.96004123392021157, -79.78289277550334191 ) ) ;
#8278=ORIENTED_EDGE ( 'NONE', *, *, #5377, .T. ) ;
#8329=VERTEX_POINT ( 'NONE', #8276 ) ;
#8332=LINE ( 'NONE', #27540, #4713 ) ;
#8338=( NAMED_UNIT ( * ) SI_UNIT ( $, .STERADIAN. ) SOLID_ANGLE_UNIT ( ) );
#8393=CARTESIAN_POINT ( 'NONE',  ( 4.440892098500000496E-16, -0.1455297029551360921, -71.05965357398815740 ) ) ;
#8409=EDGE_CURVE ( 'NONE', #6473, #10428, #12038, .T. ) ;
#8436=DIRECTION ( 'NONE',  ( 0.000000000000000000, 0.3420201433259318913, -0.9396926207858126157 ) ) ;
#8457=ORIENTED_EDGE ( 'NONE', *, *, #30368, .F. ) ;
#8494=ORIENTED_EDGE ( 'NONE', *, *, #19106, .F. ) ;
#8497=SHAPE_REPRESENTATION_RELATIONSHIP ( 'NONE' , 'NONE' ,  #6935, #9916 ) ;
#8498=VECTOR ( 'NONE', #17187, 1000.000000000000000 ) ;
#8529=ORIENTED_EDGE ( 'NONE', *, *, #3810, .F. ) ;
#8542=DIRECTION ( 'NONE',  ( -1.000000000000000000, 0.000000000000000000, 0.000000000000000000 ) ) ;
#8593=EDGE_CURVE ( 'NONE', #16796, #21922, #26793, .T. ) ;
#8607=VERTEX_POINT ( 'NONE', #16612 ) ;
#8610=EDGE_CURVE ( 'NONE', #7544, #22213, #4848, .T. ) ;
#8639=CARTESIAN_POINT ( 'NONE',  ( -9.599333685411828299, -15.14023671560908646, -74.38892505318962378 ) ) ;
#8641=VERTEX_POINT ( 'NONE', #30787 ) ;
#8646=ORIENTED_EDGE ( 'NONE', *, *, #15294, .T. ) ;
#8652=EDGE_LOOP ( 'NONE', ( #20799, #1939, #20934, #22526 ) ) ;
#8708=ORIENTED_EDGE ( 'NONE', *, *, #21800, .T. ) ;
#8728=VECTOR ( 'NONE', #16661, 1000.000000000000114 ) ;
#8735=DIRECTION ( 'NONE',  ( 0.000000000000000000, 0.3420201433259318913, -0.9396926207858126157 ) ) ;
#8746=DIRECTION ( 'NONE',  ( 0.000000000000000000, -0.3420201433259318358, 0.9396926207858125046 ) ) ;
#8753=EDGE_CURVE ( 'NONE', #18996, #18573, #27504, .T. ) ;
#8756=CYLINDRICAL_SURFACE ( 'NONE', #933, 2.000000000000003553 ) ;
#8827=ADVANCED_FACE ( 'NONE', ( #4990 ), #28744, .F. ) ;
#8830=CARTESIAN_POINT ( 'NONE',  ( 11.50000000000000000, 22.40709319595134730, -62.85117013414870257 ) ) ;
#8926=DIRECTION ( 'NONE',  ( -1.000000000000000000, 0.000000000000000000, 0.000000000000000000 ) ) ;
#8951=DIRECTION ( 'NONE',  ( 0.000000000000000000, 0.3420201433259318358, -0.9396926207858125046 ) ) ;
#8984=VECTOR ( 'NONE', #15530, 1000.000000000000000 ) ;
#9000=CARTESIAN_POINT ( 'NONE',  ( 0.6731456005949999488, -4.118494162357343669, -70.37733883405731206 ) ) ;
#9001=VERTEX_POINT ( 'NONE', #23229 ) ;
#9019=CARTESIAN_POINT ( 'NONE',  ( 6.000000000000000000, -15.86465192213301556, -74.65259062561435144 ) ) ;
#9037=LINE ( 'NONE', #18634, #7130 ) ;
#9042=DIRECTION ( 'NONE',  ( 0.7071067811780483714, -0.6644630243965946592, -0.2418447626510653037 ) ) ;
#9047=STYLED_ITEM ( 'NONE', ( #1023 ), #941 ) ;
#9088=ORIENTED_EDGE ( 'NONE', *, *, #1567, .T. ) ;
#9097=DIRECTION ( 'NONE',  ( 0.000000000000000000, 0.9396926207858125046, 0.3420201433259318358 ) ) ;
#9116=DIRECTION ( 'NONE',  ( 0.000000000000000000, 0.3420201433259318358, -0.9396926207858125046 ) ) ;
#9118=CARTESIAN_POINT ( 'NONE',  ( 4.000000000000000000, -31.83942647549183746, -80.46693306215520636 ) ) ;
#9128=VERTEX_POINT ( 'NONE', #29326 ) ;
#9193=FACE_OUTER_BOUND ( 'NONE', #7431, .T. ) ;
#9198=CARTESIAN_POINT ( 'NONE',  ( 10.00000000000000000, -13.98526668056139144, -73.96855033896248699 ) ) ;
#9238=VERTEX_POINT ( 'NONE', #24305 ) ;
#9272=CARTESIAN_POINT ( 'NONE',  ( 4.644419429734489846, -31.74345175796718621, -80.43200112173411753 ) ) ;
#9296=CARTESIAN_POINT ( 'NONE',  ( -8.000000000050000892, -13.98526668056139144, -73.96855033896248699 ) ) ;
#9341=DIRECTION ( 'NONE',  ( -0.7071067811780483714, -0.6644630243965946592, -0.2418447626510653037 ) ) ;
#9345=DIRECTION ( 'NONE',  ( 0.000000000000000000, 0.3420201433259318358, -0.9396926207858125046 ) ) ;
#9368=CARTESIAN_POINT ( 'NONE',  ( -13.00000000000000000, 24.54213077165692525, -59.94572446259928711 ) ) ;
#9430=VECTOR ( 'NONE', #22042, 1000.000000000000114 ) ;
#9472=VECTOR ( 'NONE', #8746, 1000.000000000000114 ) ;
#9491=DIRECTION ( 'NONE',  ( 0.000000000000000000, 0.3420201433259318358, -0.9396926207858125046 ) ) ;
#9536=CLOSED_SHELL ( 'NONE', ( #11922, #13086, #20326, #21579, #28663, #12544, #27756, #8827, #20360, #7326, #5192, #1986, #21551, #18954, #7797, #15699, #4836, #8231, #16394, #16321, #11428, #16379, #20542, #787, #14379, #20026, #24147, #10812, #4709, #2817, #18229, #21027, #17201, #15987, #22522, #28514, #13872, #29048, #11336, #5654, #22101, #30746 ) ) ;
#9547=FACE_OUTER_BOUND ( 'NONE', #19408, .T. ) ;
#9633=ORIENTED_EDGE ( 'NONE', *, *, #26033, .T. ) ;
#9635=ORIENTED_EDGE ( 'NONE', *, *, #17759, .T. ) ;
#9644=CARTESIAN_POINT ( 'NONE',  ( 6.000000000000000000, -29.27600094726834712, -81.66227801707495360 ) ) ;
#9646=DIRECTION ( 'NONE',  ( -0.9831920802501790124, 0.1715636151751586680, 0.06244404920691486172 ) ) ;
#9695=CARTESIAN_POINT ( 'NONE',  ( -5.747616903875187866, -30.90662447469063778, -80.12742089939932555 ) ) ;
#9702=CARTESIAN_POINT ( 'NONE',  ( -6.050735318990731137, -17.25475041001947574, -75.15854509790392513 ) ) ;
#9713=EDGE_LOOP ( 'NONE', ( #5064, #6273, #25106, #4418 ) ) ;
#9746=CARTESIAN_POINT ( 'NONE',  ( 1.346291201779999946, -3.434453875705480108, -72.25672407562892374 ) ) ;
#9751=ORIENTED_EDGE ( 'NONE', *, *, #8593, .F. ) ;
#9768=ORIENTED_EDGE ( 'NONE', *, *, #20716, .T. ) ;
#9769=VECTOR ( 'NONE', #20978, 1000.000000000000114 ) ;
#9859=CARTESIAN_POINT ( 'NONE',  ( 10.00000000000000000, -15.86465192213301556, -74.65259062561435144 ) ) ;
#9889=LINE ( 'NONE', #148, #1608 ) ;
#9897=EDGE_CURVE ( 'NONE', #25829, #18513, #14340, .T. ) ;
#9903=ORIENTED_EDGE ( 'NONE', *, *, #8409, .T. ) ;
#9916=ADVANCED_BREP_SHAPE_REPRESENTATION ( '', ( #941, #17722 ), #2296 ) ;
#9947=CARTESIAN_POINT ( 'NONE',  ( 9.414213562409999625, -15.31419272936388687, -74.45223986426802298 ) ) ;
#9955=VECTOR ( 'NONE', #10147, 1000.000000000000000 ) ;
#9957=EDGE_CURVE ( 'NONE', #1677, #18573, #19201, .T. ) ;
#10001=UNCERTAINTY_MEASURE_WITH_UNIT (LENGTH_MEASURE( 1.000000000000000082E-05 ), #15439, 'distance_accuracy_value', 'NONE');
#10033=CARTESIAN_POINT ( 'NONE',  ( -8.881784197000000993E-16, 3.378317624991660661, -69.77707803651591689 ) ) ;
#10088=CARTESIAN_POINT ( 'NONE',  ( -6.992667155225802844, -16.10181445525363841, -74.73891072835350258 ) ) ;
#10090=CARTESIAN_POINT ( 'NONE',  ( 8.000000000000000000, -15.86465192213301556, -74.65259062561435144 ) ) ;
#10091=CARTESIAN_POINT ( 'NONE',  ( 5.999999999999999112, -30.20957738316099395, -79.87371650620046637 ) ) ;
#10109=FILL_AREA_STYLE ('',( #526 ) ) ;
#10122=CARTESIAN_POINT ( 'NONE',  ( -12.94794535325927676, 25.03405588289514938, -59.76667836462032568 ) ) ;
#10147=DIRECTION ( 'NONE',  ( 1.000000000000000000, -0.000000000000000000, 0.000000000000000000 ) ) ;
#10148=VECTOR ( 'NONE', #21684, 1000.000000000000114 ) ;
#10158=CIRCLE ( 'NONE', #24239, 2.000000000000000000 ) ;
#10219=VERTEX_POINT ( 'NONE', #26823 ) ;
#10233=LINE ( 'NONE', #29726, #2540 ) ;
#10247=AXIS2_PLACEMENT_3D ( 'NONE', #30999, #6028, #20672 ) ;
#10258=DIRECTION ( 'NONE',  ( 0.000000000000000000, 0.3420201433259318358, -0.9396926207858125046 ) ) ;
#10280=CARTESIAN_POINT ( 'NONE',  ( 0.000000000000000000, 4.811145170119999648, -67.12721591429999535 ) ) ;
#10294=VECTOR ( 'NONE', #22247, 1000.000000000000114 ) ;
#10296=EDGE_CURVE ( 'NONE', #21919, #9128, #24013, .T. ) ;
#10381=DIRECTION ( 'NONE',  ( 0.000000000000000000, 0.9396926207858125046, 0.3420201433259318358 ) ) ;
#10394=DIRECTION ( 'NONE',  ( -1.000000000000000000, 0.000000000000000000, 0.000000000000000000 ) ) ;
#10406=DIRECTION ( 'NONE',  ( 0.000000000000000000, -0.3420201433259318913, 0.9396926207858126157 ) ) ;
#10428=VERTEX_POINT ( 'NONE', #6659 ) ;
#10479=VECTOR ( 'NONE', #13479, 1000.000000000000114 ) ;
#10481=DIRECTION ( 'NONE',  ( 0.000000000000000000, 0.3420201433259318358, -0.9396926207858125046 ) ) ;
#10490=CARTESIAN_POINT ( 'NONE',  ( -8.000000000050000892, -13.30122639390952877, -75.84793558053411289 ) ) ;
#10498=ORIENTED_EDGE ( 'NONE', *, *, #25956, .F. ) ;
#10543=CARTESIAN_POINT ( 'NONE',  ( -13.00000000000000000, 22.40709319595134730, -62.85117013414870257 ) ) ;
#10570=ORIENTED_EDGE ( 'NONE', *, *, #21058, .T. ) ;
#10628=FACE_OUTER_BOUND ( 'NONE', #16360, .T. ) ;
#10630=VECTOR ( 'NONE', #4440, 1000.000000000000114 ) ;
#10649=VECTOR ( 'NONE', #24413, 1000.000000000000000 ) ;
#10659=CARTESIAN_POINT ( 'NONE',  ( 8.000000000000000000, -17.05999687705277879, -77.21601615383784178 ) ) ;
#10695=CARTESIAN_POINT ( 'NONE',  ( -6.000000000000000000, -23.16799891216055940, -79.43914708545641190 ) ) ;
#10705=CARTESIAN_POINT ( 'NONE',  ( -5.414213562369999622, -31.28896728272270877, -80.26658230080884948 ) ) ;
#10747=VECTOR ( 'NONE', #2920, 1000.000000000000000 ) ;
#10754=CIRCLE ( 'NONE', #24329, 2.000000000000000000 ) ;
#10764=SURFACE_STYLE_FILL_AREA ( #22580 ) ;
#10774=CIRCLE ( 'NONE', #20343, 2.000000000000000000 ) ;
#10812=ADVANCED_FACE ( 'NONE', ( #7699 ), #8004, .T. ) ;
#10822=CARTESIAN_POINT ( 'NONE',  ( -8.000000000000000000, -17.74403716370463968, -75.33663091226621589 ) ) ;
#10856=VERTEX_POINT ( 'NONE', #645 ) ;
#10873=CARTESIAN_POINT ( 'NONE',  ( -5.010133801301174472, -31.60104845553905761, -80.38017055838898273 ) ) ;
#10919=CARTESIAN_POINT ( 'NONE',  ( 0.000000000000000000, 5.495185456771864096, -69.00660115587162124 ) ) ;
#10955=EDGE_CURVE ( 'NONE', #31086, #7075, #4383, .T. ) ;
#10977=B_SPLINE_CURVE_WITH_KNOTS ( 'NONE', 3,
 ( #22056, #507, #39, #7265, #10091, #19685 ),
 .UNSPECIFIED., .F., .F.,
 ( 4, 2, 4 ),
 ( 0.000000000000000000, 0.5000000000000000000, 1.000000000000000000 ),
 .UNSPECIFIED. ) ;
#11066=VERTEX_POINT ( 'NONE', #21848 ) ;
#11088=CARTESIAN_POINT ( 'NONE',  ( 4.000000000000000000, -31.83942647549183746, -80.46693306215520636 ) ) ;
#11092=ORIENTED_EDGE ( 'NONE', *, *, #3075, .F. ) ;
#11115=VERTEX_POINT ( 'NONE', #12858 ) ;
#11124=CARTESIAN_POINT ( 'NONE',  ( 6.585786437629999490, -16.41511111490214603, -74.85294138696069410 ) ) ;
#11129=CARTESIAN_POINT ( 'NONE',  ( 3.059320232295363873, -2.907977535978094163, -69.93674681397055792 ) ) ;
#11156=CARTESIAN_POINT ( 'NONE',  ( 1.243449787579999883E-14, -31.15538618883996946, -82.34631830372681804 ) ) ;
#11185=ORIENTED_EDGE ( 'NONE', *, *, #19483, .F. ) ;
#11226=ORIENTED_EDGE ( 'NONE', *, *, #16574, .F. ) ;
#11252=FACE_OUTER_BOUND ( 'NONE', #5353, .T. ) ;
#11271=EDGE_LOOP ( 'NONE', ( #8708, #132, #28775, #11344 ) ) ;
#11277=AXIS2_PLACEMENT_3D ( 'NONE', #14206, #12305, #2254 ) ;
#11279=CARTESIAN_POINT ( 'NONE',  ( -13.00000000000000000, 21.72305290929948640, -60.97178489257708378 ) ) ;
#11305=ORIENTED_EDGE ( 'NONE', *, *, #29371, .F. ) ;
#11336=ADVANCED_FACE ( 'NONE', ( #12158 ), #7743, .F. ) ;
#11344=ORIENTED_EDGE ( 'NONE', *, *, #19314, .F. ) ;
#11345=ORIENTED_EDGE ( 'NONE', *, *, #14233, .T. ) ;
#11363=EDGE_CURVE ( 'NONE', #5989, #10856, #1999, .T. ) ;
#11365=CARTESIAN_POINT ( 'NONE',  ( 6.000000000000000000, -29.96004123392021157, -79.78289277550334191 ) ) ;
#11374=ORIENTED_EDGE ( 'NONE', *, *, #6563, .T. ) ;
#11428=ADVANCED_FACE ( 'NONE', ( #16880 ), #14849, .F. ) ;
#11465=VECTOR ( 'NONE', #2433, 1000.000000000000000 ) ;
#11508=VECTOR ( 'NONE', #1694, 1000.000000000000114 ) ;
#11526=ORIENTED_EDGE ( 'NONE', *, *, #22370, .T. ) ;
#11538=ORIENTED_EDGE ( 'NONE', *, *, #8753, .T. ) ;
#11574=CARTESIAN_POINT ( 'NONE',  ( 3.015246714024014452, 1.304698913893802104, -68.40345797962162067 ) ) ;
#11575=CARTESIAN_POINT ( 'NONE',  ( 9.599333684284403034, -15.14023671706337915, -74.38892505371892128 ) ) ;
#11588=PRODUCT_DEFINITION_CONTEXT ( 'detailed design', #544, 'design' ) ;
#11663=DIRECTION ( 'NONE',  ( 0.7071067811780481493, 0.6644630243965948813, 0.2418447626510653869 ) ) ;
#11675=DIRECTION ( 'NONE',  ( 0.000000000000000000, 0.9396926207858125046, 0.3420201433259318358 ) ) ;
#11706=FACE_OUTER_BOUND ( 'NONE', #16673, .T. ) ;
#11728=VECTOR ( 'NONE', #24983, 1000.000000000000114 ) ;
#11730=ORIENTED_EDGE ( 'NONE', *, *, #30355, .F. ) ;
#11739=CARTESIAN_POINT ( 'NONE',  ( -12.59933368422367472, 25.69710080817275255, -59.52534974783780086 ) ) ;
#11765=VECTOR ( 'NONE', #10481, 1000.000000000000114 ) ;
#11790=DIRECTION ( 'NONE',  ( 0.000000000000000000, 0.3420201433259318913, -0.9396926207858126157 ) ) ;
#11820=EDGE_CURVE ( 'NONE', #13699, #29409, #13972, .T. ) ;
#11902=DIRECTION ( 'NONE',  ( 0.000000000000000000, 0.9396926207858125046, 0.3420201433259318358 ) ) ;
#11922=ADVANCED_FACE ( 'NONE', ( #15065 ), #21999, .T. ) ;
#11950=CARTESIAN_POINT ( 'NONE',  ( 6.000000000000000000, -17.74403716370463968, -75.33663091226621589 ) ) ;
#11966=CARTESIAN_POINT ( 'NONE',  ( -12.41421356240000051, 26.55509710711128335, -61.34142017886538412 ) ) ;
#12002=CIRCLE ( 'NONE', #476, 2.000000000000000000 ) ;
#12011=ORIENTED_EDGE ( 'NONE', *, *, #16712, .T. ) ;
#12038=B_SPLINE_CURVE_WITH_KNOTS ( 'NONE', 3,
 ( #1533, #18026, #30156, #20887, #13476, #11124 ),
 .UNSPECIFIED., .F., .F.,
 ( 4, 2, 4 ),
 ( 0.000000000000000000, 0.5000000000000000000, 1.000000000000000000 ),
 .UNSPECIFIED. ) ;
#12087=VERTEX_POINT ( 'NONE', #11279 ) ;
#12158=FACE_OUTER_BOUND ( 'NONE', #20008, .T. ) ;
#12164=DIRECTION ( 'NONE',  ( -0.000000000000000000, -0.9396926207858126157, -0.3420201433259318913 ) ) ;
#12166=DIRECTION ( 'NONE',  ( 0.000000000000000000, 0.3420201433259318913, -0.9396926207858126157 ) ) ;
#12189=EDGE_CURVE ( 'NONE', #11066, #9001, #30637, .T. ) ;
#12208=DIRECTION ( 'NONE',  ( -0.000000000000000000, -0.9396926207858126157, -0.3420201433259318913 ) ) ;
#12212=FACE_OUTER_BOUND ( 'NONE', #19547, .T. ) ;
#12292=CARTESIAN_POINT ( 'NONE',  ( -10.00000000000000000, 22.40709319595134730, -62.85117013414870257 ) ) ;
#12298=ORIENTED_EDGE ( 'NONE', *, *, #22370, .F. ) ;
#12305=DIRECTION ( 'NONE',  ( 0.000000000000000000, 0.3420201433259318913, -0.9396926207858126157 ) ) ;
#12353=DIRECTION ( 'NONE',  ( 0.000000000000000000, 0.9396926207858125046, 0.3420201433259318358 ) ) ;
#12355=DIRECTION ( 'NONE',  ( -0.7071067811865475727, 0.6644630243886071597, 0.2418447626481610435 ) ) ;
#12373=CARTESIAN_POINT ( 'NONE',  ( -0.6731456005949999488, -4.118494162357343669, -70.37733883405731206 ) ) ;
#12374=EDGE_CURVE ( 'NONE', #22213, #18513, #14036, .T. ) ;
#12375=ORIENTED_EDGE ( 'NONE', *, *, #27306, .F. ) ;
#12381=DIRECTION ( 'NONE',  ( 1.000000000000000000, 0.000000000000000000, 0.000000000000000000 ) ) ;
#12396=ORIENTED_EDGE ( 'NONE', *, *, #28404, .F. ) ;
#12400=CARTESIAN_POINT ( 'NONE',  ( 2.553512956640000223E-15, 3.378317624991660661, -69.77707803651591689 ) ) ;
#12405=CARTESIAN_POINT ( 'NONE',  ( 4.000000000000000000, -29.96004123392021157, -79.78289277550334191 ) ) ;
#12431=DIRECTION ( 'NONE',  ( -1.000000000000000000, -0.000000000000000000, 0.000000000000000000 ) ) ;
#12496=ORIENTED_EDGE ( 'NONE', *, *, #27071, .T. ) ;
#12544=ADVANCED_FACE ( 'NONE', ( #23482 ), #1918, .F. ) ;
#12588=CARTESIAN_POINT ( 'NONE',  ( -6.585786437629999490, -16.41511111490214603, -74.85294138696069410 ) ) ;
#12598=CARTESIAN_POINT ( 'NONE',  ( -5.414213562369999622, -31.28896728272270877, -80.26658230080884948 ) ) ;
#12699=EDGE_CURVE ( 'NONE', #25829, #22642, #29789, .T. ) ;
#12723=ORIENTED_EDGE ( 'NONE', *, *, #11363, .F. ) ;
#12730=B_SPLINE_CURVE_WITH_KNOTS ( 'NONE', 3,
 ( #26395, #28739, #7188, #9702, #14434, #19149 ),
 .UNSPECIFIED., .F., .F.,
 ( 4, 2, 4 ),
 ( 0.000000000000000000, 0.5000000000000000000, 1.000000000000000000 ),
 .UNSPECIFIED. ) ;
#12731=LINE ( 'NONE', #5345, #26620 ) ;
#12757=CARTESIAN_POINT ( 'NONE',  ( -4.265551103502377650, -31.83942647549183746, -80.46693306215522057 ) ) ;
#12771=AXIS2_PLACEMENT_3D ( 'NONE', #1661, #30920, #9042 ) ;
#12828=ORIENTED_EDGE ( 'NONE', *, *, #8593, .T. ) ;
#12858=CARTESIAN_POINT ( 'NONE',  ( 9.414213562409999625, -14.63015244271202420, -76.33162510583964888 ) ) ;
#12880=ORIENTED_EDGE ( 'NONE', *, *, #13840, .F. ) ;
#12897=DIRECTION ( 'NONE',  ( 0.000000000000000000, 0.3420201433259318358, -0.9396926207858125046 ) ) ;
#12969=SURFACE_SIDE_STYLE ('',( #10764 ) ) ;
#13009=FACE_OUTER_BOUND ( 'NONE', #30295, .T. ) ;
#13010=EDGE_LOOP ( 'NONE', ( #29599, #3162, #26936, #5747 ) ) ;
#13016=DIRECTION ( 'NONE',  ( 0.000000000000000000, -0.3420201433259318913, 0.9396926207858126157 ) ) ;
#13078=DIRECTION ( 'NONE',  ( 0.000000000000000000, 0.3420201433259318913, -0.9396926207858126157 ) ) ;
#13086=ADVANCED_FACE ( 'NONE', ( #13009 ), #14266, .T. ) ;
#13104=ORIENTED_EDGE ( 'NONE', *, *, #6563, .F. ) ;
#13117=( NAMED_UNIT ( * ) SI_UNIT ( $, .STERADIAN. ) SOLID_ANGLE_UNIT ( ) );
#13205=CARTESIAN_POINT ( 'NONE',  ( -9.414213562409999625, -15.31419272936388687, -74.45223986426802298 ) ) ;
#13233=AXIS2_PLACEMENT_3D ( 'NONE', #6484, #18442, #30722 ) ;
#13251=ORIENTED_EDGE ( 'NONE', *, *, #10955, .F. ) ;
#13256=DIRECTION ( 'NONE',  ( 1.000000000000000000, -0.000000000000000000, 0.000000000000000000 ) ) ;
#13327=CARTESIAN_POINT ( 'NONE',  ( -7.355580493362803729, -15.96062638079863483, -74.68752247181846826 ) ) ;
#13372=DIRECTION ( 'NONE',  ( 0.000000000000000000, 0.3420201433259318358, -0.9396926207858125046 ) ) ;
#13375=VERTEX_POINT ( 'NONE', #19137 ) ;
#13380=CARTESIAN_POINT ( 'NONE',  ( 4.000000000000000000, -31.15538618883996946, -82.34631830372681804 ) ) ;
#13382=EDGE_LOOP ( 'NONE', ( #19660, #19584, #29804, #7503 ) ) ;
#13390=DIRECTION ( 'NONE',  ( 1.000000000000000000, -0.000000000000000000, 0.000000000000000000 ) ) ;
#13440=ORIENTED_EDGE ( 'NONE', *, *, #23883, .T. ) ;
#13463=ORIENTED_EDGE ( 'NONE', *, *, #1567, .F. ) ;
#13476=CARTESIAN_POINT ( 'NONE',  ( 6.770906559283583981, -16.24115510245209038, -74.78962657635717903 ) ) ;
#13479=DIRECTION ( 'NONE',  ( 0.000000000000000000, -0.3420201433259318358, 0.9396926207858125046 ) ) ;
#13481=EDGE_CURVE ( 'NONE', #24619, #8103, #29962, .T. ) ;
#13500=AXIS2_PLACEMENT_3D ( 'NONE', #30165, #3414, #18198 ) ;
#13533=CARTESIAN_POINT ( 'NONE',  ( 11.00000000000000000, 26.42151601322854759, -59.26168417594741555 ) ) ;
#13542=ORIENTED_EDGE ( 'NONE', *, *, #23342, .T. ) ;
#13543=( NAMED_UNIT ( * ) SI_UNIT ( $, .STERADIAN. ) SOLID_ANGLE_UNIT ( ) );
#13568=LINE ( 'NONE', #11365, #10630 ) ;
#13589=ORIENTED_EDGE ( 'NONE', *, *, #1528, .F. ) ;
#13655=CARTESIAN_POINT ( 'NONE',  ( 0.000000000000000000, 21.72305290929948640, -60.97178489257708378 ) ) ;
#13699=VERTEX_POINT ( 'NONE', #19569 ) ;
#13718=DIRECTION ( 'NONE',  ( -0.000000000000000000, -0.9396926207858126157, -0.3420201433259318913 ) ) ;
#13723=CARTESIAN_POINT ( 'NONE',  ( 5.414213562369999622, -30.60492699607083722, -82.14596754238048959 ) ) ;
#13767=ORIENTED_EDGE ( 'NONE', *, *, #22334, .T. ) ;
#13775=CARTESIAN_POINT ( 'NONE',  ( 1.682565990562016722, 2.345890382669250762, -68.02449527681511654 ) ) ;
#13796=DIRECTION ( 'NONE',  ( 0.000000000000000000, 0.9396926207858125046, 0.3420201433259318358 ) ) ;
#13823=ORIENTED_EDGE ( 'NONE', *, *, #13910, .T. ) ;
#13828=LINE ( 'NONE', #19006, #26244 ) ;
#13838=DIRECTION ( 'NONE',  ( -0.000000000000000000, -0.9396926207858126157, -0.3420201433259318913 ) ) ;
#13840=EDGE_CURVE ( 'NONE', #8329, #8607, #8201, .T. ) ;
#13856=CARTESIAN_POINT ( 'NONE',  ( -8.000000000050000892, -13.30122639390952877, -75.84793558053411289 ) ) ;
#13861=ORIENTED_EDGE ( 'NONE', *, *, #23979, .T. ) ;
#13872=ADVANCED_FACE ( 'NONE', ( #15455 ), #20178, .F. ) ;
#13897=B_SPLINE_CURVE_WITH_KNOTS ( 'NONE', 3,
 ( #16664, #16361, #23928, #28776, #2365, #11950 ),
 .UNSPECIFIED., .F., .F.,
 ( 4, 2, 4 ),
 ( 0.000000000000000000, 0.5000000000000000000, 1.000000000000000000 ),
 .UNSPECIFIED. ) ;
#13900=CARTESIAN_POINT ( 'NONE',  ( -7.000000000000000000, -15.86465192213301556, -74.65259062561435144 ) ) ;
#13906=PLANE ( 'NONE',  #3396 ) ;
#13910=EDGE_CURVE ( 'NONE', #29055, #17565, #6327, .T. ) ;
#13925=DIRECTION ( 'NONE',  ( 0.000000000000000000, 0.3420201433259318358, -0.9396926207858125046 ) ) ;
#13972=CIRCLE ( 'NONE', #20029, 2.000000000000000000 ) ;
#14015=DIRECTION ( 'NONE',  ( 0.000000000000000000, 0.000000000000000000, 1.000000000000000000 ) ) ;
#14031=AXIS2_PLACEMENT_3D ( 'NONE', #10280, #25057, #27261 ) ;
#14036=B_SPLINE_CURVE_WITH_KNOTS ( 'NONE', 3,
 ( #3636, #3961, #25686, #15754, #17945, #29763 ),
 .UNSPECIFIED., .F., .F.,
 ( 4, 2, 4 ),
 ( 0.000000000000000000, 0.5000000000000000000, 1.000000000000000000 ),
 .UNSPECIFIED. ) ;
#14059=VERTEX_POINT ( 'NONE', #7827 ) ;
#14100=EDGE_LOOP ( 'NONE', ( #2145, #30663, #24232, #9768 ) ) ;
#14109=B_SPLINE_CURVE_WITH_KNOTS ( 'NONE', 3,
 ( #10705, #3156, #10873, #29905, #12757, #3462 ),
 .UNSPECIFIED., .F., .F.,
 ( 4, 2, 4 ),
 ( 0.000000000000000000, 0.5000000000000000000, 1.000000000000000000 ),
 .UNSPECIFIED. ) ;
#14110=DIRECTION ( 'NONE',  ( 0.000000000000000000, 0.3420201433259318358, -0.9396926207858125046 ) ) ;
#14206=CARTESIAN_POINT ( 'NONE',  ( 0.000000000000000000, 4.811145170119999648, -67.12721591429999535 ) ) ;
#14209=EDGE_LOOP ( 'NONE', ( #21214, #12011, #13861, #8494 ) ) ;
#14226=PLANE ( 'NONE',  #18361 ) ;
#14230=CARTESIAN_POINT ( 'NONE',  ( -8.000000000050000892, -13.98526668056139144, -73.96855033896248699 ) ) ;
#14233=EDGE_CURVE ( 'NONE', #26031, #23194, #24978, .T. ) ;
#14258=EDGE_CURVE ( 'NONE', #10219, #18996, #12002, .T. ) ;
#14266=PLANE ( 'NONE',  #7975 ) ;
#14288=CARTESIAN_POINT ( 'NONE',  ( 8.000000000000000000, -17.05999687705277879, -77.21601615383784178 ) ) ;
#14330=CIRCLE ( 'NONE', #759, 3.750000000000000000 ) ;
#14340=LINE ( 'NONE', #28486, #7940 ) ;
#14370=PLANE ( 'NONE',  #11277 ) ;
#14373=ORIENTED_EDGE ( 'NONE', *, *, #18727, .T. ) ;
#14379=ADVANCED_FACE ( 'NONE', ( #15380 ), #30002, .F. ) ;
#14381=DIRECTION ( 'NONE',  ( -1.000000000000000000, 0.000000000000000000, 0.000000000000000000 ) ) ;
#14434=CARTESIAN_POINT ( 'NONE',  ( -6.000000000000000000, -17.49450075019272433, -75.24580708538225338 ) ) ;
#14447=EDGE_CURVE ( 'NONE', #23530, #25602, #19144, .T. ) ;
#14477=ORIENTED_EDGE ( 'NONE', *, *, #30355, .T. ) ;
#14527=EDGE_CURVE ( 'NONE', #8329, #29142, #30465, .T. ) ;
#14528=VECTOR ( 'NONE', #26114, 1000.000000000000114 ) ;
#14534=CARTESIAN_POINT ( 'NONE',  ( -10.00000000000000000, -13.64324653723545921, -74.90824295974830704 ) ) ;
#14536=CARTESIAN_POINT ( 'NONE',  ( 8.000000000000000000, -17.74403716370463968, -75.33663091226621589 ) ) ;
#14549=LINE ( 'NONE', #22092, #11465 ) ;
#14555=EDGE_CURVE ( 'NONE', #3795, #7075, #26536, .T. ) ;
#14567=ORIENTED_EDGE ( 'NONE', *, *, #10296, .T. ) ;
#14575=FACE_OUTER_BOUND ( 'NONE', #23245, .T. ) ;
#14580=ORIENTED_EDGE ( 'NONE', *, *, #22334, .F. ) ;
#14619=DIRECTION ( 'NONE',  ( 0.000000000000000000, 0.3420201433259318358, -0.9396926207858125046 ) ) ;
#14654=CARTESIAN_POINT ( 'NONE',  ( 13.00000000000000000, 23.81663212713006672, -62.33813991915980779 ) ) ;
#14659=CARTESIAN_POINT ( 'NONE',  ( -8.000000000000000000, -15.86465192213301556, -74.65259062561435144 ) ) ;
#14733=DIRECTION ( 'NONE',  ( 0.000000000000000000, 0.3420201433259318358, -0.9396926207858125046 ) ) ;
#14744=DIRECTION ( 'NONE',  ( -0.7071067811865467956, -0.6644630243886068266, -0.2418447626481644297 ) ) ;
#14748=DIRECTION ( 'NONE',  ( -1.000000000000000000, 0.000000000000000000, 0.000000000000000000 ) ) ;
#14752=CARTESIAN_POINT ( 'NONE',  ( 13.00000000000000000, 21.72305290929948640, -60.97178489257708378 ) ) ;
#14770=DIRECTION ( 'NONE',  ( 0.7071067811865467956, -0.6644630243886068266, -0.2418447626481644297 ) ) ;
#14791=SHAPE_DEFINITION_REPRESENTATION ( #30767, #6935 ) ;
#14849=CYLINDRICAL_SURFACE ( 'NONE', #1912, 3.749999999999999556 ) ;
#14934=EDGE_CURVE ( 'NONE', #19754, #9128, #14549, .T. ) ;
#14961=CARTESIAN_POINT ( 'NONE',  ( -7.482225056410205077, -15.92425073469576979, -74.67428281938484247 ) ) ;
#14972=CARTESIAN_POINT ( 'NONE',  ( 6.339027081030000540E-10, -4.118494162357343669, -70.37733883405731206 ) ) ;
#14977=DIRECTION ( 'NONE',  ( -1.000000000000000000, 0.000000000000000000, 0.000000000000000000 ) ) ;
#14979=ORIENTED_EDGE ( 'NONE', *, *, #18525, .F. ) ;
#14982=CARTESIAN_POINT ( 'NONE',  ( 10.00000000005000267, -14.23127763357968156, -74.05809100316466242 ) ) ;
#14983=ORIENTED_EDGE ( 'NONE', *, *, #23382, .T. ) ;
#14996=ORIENTED_EDGE ( 'NONE', *, *, #1892, .F. ) ;
#15036=CARTESIAN_POINT ( 'NONE',  ( 4.440892098500000496E-16, -0.1455297029551360921, -71.05965357398815740 ) ) ;
#15040=DIRECTION ( 'NONE',  ( 0.000000000000000000, -0.3420201433259318913, 0.9396926207858126157 ) ) ;
#15065=FACE_OUTER_BOUND ( 'NONE', #21897, .T. ) ;
#15160=EDGE_CURVE ( 'NONE', #22213, #29409, #4574, .T. ) ;
#15165=ORIENTED_EDGE ( 'NONE', *, *, #7689, .T. ) ;
#15180=AXIS2_PLACEMENT_3D ( 'NONE', #27147, #15040, #267 ) ;
#15190=CARTESIAN_POINT ( 'NONE',  ( -9.414213562409999625, -15.31419272936388687, -74.45223986426802298 ) ) ;
#15227=CARTESIAN_POINT ( 'NONE',  ( 6.000000000000000000, -15.18061163548115466, -76.53197586718597734 ) ) ;
#15272=LINE ( 'NONE', #6131, #27820 ) ;
#15294=EDGE_CURVE ( 'NONE', #26555, #24268, #29106, .T. ) ;
#15311=DIRECTION ( 'NONE',  ( -1.000000000000000000, 0.000000000000000000, 0.000000000000000000 ) ) ;
#15358=ORIENTED_EDGE ( 'NONE', *, *, #25806, .F. ) ;
#15380=FACE_OUTER_BOUND ( 'NONE', #4102, .T. ) ;
#15387=EDGE_CURVE ( 'NONE', #19754, #18573, #27290, .T. ) ;
#15409=CARTESIAN_POINT ( 'NONE',  ( -11.00000000000000000, 26.42151601322854759, -59.26168417594741555 ) ) ;
#15436=VERTEX_POINT ( 'NONE', #11088 ) ;
#15439=( LENGTH_UNIT ( ) NAMED_UNIT ( * ) SI_UNIT ( .MILLI., .METRE. ) );
#15444=LINE ( 'NONE', #18258, #26892 ) ;
#15455=FACE_OUTER_BOUND ( 'NONE', #1597, .T. ) ;
#15473=ORIENTED_EDGE ( 'NONE', *, *, #1892, .T. ) ;
#15474=VERTEX_POINT ( 'NONE', #29576 ) ;
#15530=DIRECTION ( 'NONE',  ( -1.000000000000000000, 0.000000000000000000, 0.000000000000000000 ) ) ;
#15534=AXIS2_PLACEMENT_3D ( 'NONE', #2762, #29490, #12355 ) ;
#15556=CARTESIAN_POINT ( 'NONE',  ( 11.52349576909532303, 26.37260064581004215, -59.27948791368598336 ) ) ;
#15565=DIRECTION ( 'NONE',  ( 1.000000000000000000, -0.000000000000000000, 0.000000000000000000 ) ) ;
#15584=ORIENTED_EDGE ( 'NONE', *, *, #8610, .T. ) ;
#15587=EDGE_LOOP ( 'NONE', ( #22985, #22494, #12396, #13589, #19553, #12298, #8529, #11305, #7100, #19944 ) ) ;
#15651=LINE ( 'NONE', #25580, #11765 ) ;
#15659=CIRCLE ( 'NONE', #3103, 2.000000000000000000 ) ;
#15699=ADVANCED_FACE ( 'NONE', ( #23133 ), #6592, .F. ) ;
#15754=CARTESIAN_POINT ( 'NONE',  ( -11.52349576831824507, 26.37260064595716358, -59.27948791363240844 ) ) ;
#15759=EDGE_CURVE ( 'NONE', #6473, #10219, #30524, .T. ) ;
#15844=CARTESIAN_POINT ( 'NONE',  ( 3.686970300939999667, 0.4978338539504151838, -70.82548838946271985 ) ) ;
#15885=CARTESIAN_POINT ( 'NONE',  ( -0.6731456008920000400, -3.434453875705480108, -72.25672407562892374 ) ) ;
#15909=ORIENTED_EDGE ( 'NONE', *, *, #12189, .F. ) ;
#15934=FACE_OUTER_BOUND ( 'NONE', #2975, .T. ) ;
#15979=EDGE_CURVE ( 'NONE', #11115, #24784, #3726, .T. ) ;
#15987=ADVANCED_FACE ( 'NONE', ( #20891 ), #8756, .T. ) ;
#16000=DIRECTION ( 'NONE',  ( 0.000000000000000000, 0.3420201433259318913, -0.9396926207858126157 ) ) ;
#16001=ORIENTED_EDGE ( 'NONE', *, *, #3481, .T. ) ;
#16015=CARTESIAN_POINT ( 'NONE',  ( -6.000000000000000000, -23.16799891216055940, -79.43914708545641190 ) ) ;
#16021=ORIENTED_EDGE ( 'NONE', *, *, #15979, .F. ) ;
#16043=PLANE ( 'NONE',  #19751 ) ;
#16176=VECTOR ( 'NONE', #15565, 1000.000000000000000 ) ;
#16180=ORIENTED_EDGE ( 'NONE', *, *, #12699, .T. ) ;
#16182=EDGE_CURVE ( 'NONE', #10856, #21922, #6650, .T. ) ;
#16249=ORIENTED_EDGE ( 'NONE', *, *, #26237, .T. ) ;
#16321=ADVANCED_FACE ( 'NONE', ( #5886 ), #29964, .F. ) ;
#16324=CARTESIAN_POINT ( 'NONE',  ( -7.000000000000000000, -15.18061163548115466, -76.53197586718597734 ) ) ;
#16326=VECTOR ( 'NONE', #8926, 1000.000000000000000 ) ;
#16360=EDGE_LOOP ( 'NONE', ( #21376, #4017, #11730, #16180 ) ) ;
#16361=CARTESIAN_POINT ( 'NONE',  ( 6.400666314641494381, -16.58906712865265831, -74.91625619803754432 ) ) ;
#16363=DIRECTION ( 'NONE',  ( -1.000000000000000000, 0.000000000000000000, 0.000000000000000000 ) ) ;
#16374=ORIENTED_EDGE ( 'NONE', *, *, #27306, .T. ) ;
#16379=ADVANCED_FACE ( 'NONE', ( #16429 ), #23835, .T. ) ;
#16394=ADVANCED_FACE ( 'NONE', ( #18783 ), #28393, .F. ) ;
#16429=FACE_OUTER_BOUND ( 'NONE', #4687, .T. ) ;
#16432=LINE ( 'NONE', #17012, #20699 ) ;
#16489=DIRECTION ( 'NONE',  ( 0.000000000000000000, 0.3420201433259318913, -0.9396926207858126157 ) ) ;
#16514=CARTESIAN_POINT ( 'NONE',  ( -3.484426971583858279, -2.194289969034543208, -69.67698578303701140 ) ) ;
#16574=EDGE_CURVE ( 'NONE', #8147, #11115, #10158, .T. ) ;
#16612=CARTESIAN_POINT ( 'NONE',  ( -6.000000000000000000, -29.27600094726834712, -81.66227801707495360 ) ) ;
#16643=VECTOR ( 'NONE', #19494, 1000.000000000000114 ) ;
#16655=CARTESIAN_POINT ( 'NONE',  ( 0.000000000000000000, -15.86465192213301556, -74.65259062561435144 ) ) ;
#16661=DIRECTION ( 'NONE',  ( 0.000000000000000000, -0.9396926207858125046, -0.3420201433259318358 ) ) ;
#16664=CARTESIAN_POINT ( 'NONE',  ( 6.585786437629999490, -16.41511111490214603, -74.85294138696069410 ) ) ;
#16673=EDGE_LOOP ( 'NONE', ( #2633, #18924, #11538, #22073 ) ) ;
#16703=FACE_OUTER_BOUND ( 'NONE', #11271, .T. ) ;
#16712=EDGE_CURVE ( 'NONE', #12087, #7544, #21119, .T. ) ;
#16713=CARTESIAN_POINT ( 'NONE',  ( 8.000000000000000000, -15.86465192213301556, -74.65259062561435144 ) ) ;
#16794=ORIENTED_EDGE ( 'NONE', *, *, #4587, .T. ) ;
#16796=VERTEX_POINT ( 'NONE', #14659 ) ;
#16800=LINE ( 'NONE', #6741, #27497 ) ;
#16820=EDGE_CURVE ( 'NONE', #12087, #18533, #348, .T. ) ;
#16838=ORIENTED_EDGE ( 'NONE', *, *, #26750, .T. ) ;
#16853=( GEOMETRIC_REPRESENTATION_CONTEXT ( 3 ) GLOBAL_UNCERTAINTY_ASSIGNED_CONTEXT ( ( #24164 ) ) GLOBAL_UNIT_ASSIGNED_CONTEXT ( ( #22994, #3796, #13543 ) ) REPRESENTATION_CONTEXT ( 'NONE', 'WORKASPACE' ) );
#16864=ORIENTED_EDGE ( 'NONE', *, *, #27071, .F. ) ;
#16880=FACE_OUTER_BOUND ( 'NONE', #21446, .T. ) ;
#16929=CARTESIAN_POINT ( 'NONE',  ( -9.007237961434523044, -15.62744792279970696, -74.56625543040802029 ) ) ;
#16992=ORIENTED_EDGE ( 'NONE', *, *, #14258, .F. ) ;
#16999=EDGE_CURVE ( 'NONE', #18765, #11066, #20715, .T. ) ;
#17012=CARTESIAN_POINT ( 'NONE',  ( 10.00000000000000000, 22.06507305262541863, -61.91147751336289673 ) ) ;
#17073=CARTESIAN_POINT ( 'NONE',  ( -10.00000000000000000, 21.72305290929948640, -60.97178489257708378 ) ) ;
#17078=EDGE_LOOP ( 'NONE', ( #25392, #18449, #19235, #16794 ) ) ;
#17084=CARTESIAN_POINT ( 'NONE',  ( -5.987315253674642790, -30.20684655539371732, -79.87272256617823984 ) ) ;
#17089=DIRECTION ( 'NONE',  ( 0.000000000000000000, -0.9396926207858125046, -0.3420201433259318358 ) ) ;
#17130=ORIENTED_EDGE ( 'NONE', *, *, #14934, .T. ) ;
#17187=DIRECTION ( 'NONE',  ( 1.000000000000000000, -0.000000000000000000, 0.000000000000000000 ) ) ;
#17190=CARTESIAN_POINT ( 'NONE',  ( -12.41421356240000051, 25.87105682045942245, -59.46203493729375822 ) ) ;
#17192=CARTESIAN_POINT ( 'NONE',  ( 0.6731456008920000400, -3.434453875705480108, -72.25672407562892374 ) ) ;
#17201=ADVANCED_FACE ( 'NONE', ( #9547 ), #16043, .T. ) ;
#17205=CARTESIAN_POINT ( 'NONE',  ( 6.000000000000000000, -16.80434454291883029, -74.99461076894029077 ) ) ;
#17235=CARTESIAN_POINT ( 'NONE',  ( -5.414213562369999622, -31.28896728272270877, -80.26658230080884948 ) ) ;
#17244=VECTOR ( 'NONE', #11675, 1000.000000000000114 ) ;
#17256=DIRECTION ( 'NONE',  ( 0.000000000000000000, -0.9396926207858125046, -0.3420201433259318358 ) ) ;
#17257=VECTOR ( 'NONE', #18714, 1000.000000000000000 ) ;
#17313=VECTOR ( 'NONE', #20027, 1000.000000000000114 ) ;
#17314=CARTESIAN_POINT ( 'NONE',  ( 3.771189585364855379, -0.9962994085146968937, -69.24095287807548971 ) ) ;
#17346=EDGE_CURVE ( 'NONE', #24268, #8147, #18788, .T. ) ;
#17476=LINE ( 'NONE', #22064, #18298 ) ;
#17531=CARTESIAN_POINT ( 'NONE',  ( 11.00000000000000000, 25.22617105830878614, -61.82510970417090590 ) ) ;
#17565=VERTEX_POINT ( 'NONE', #13723 ) ;
#17573=ORIENTED_EDGE ( 'NONE', *, *, #13910, .F. ) ;
#17582=LINE ( 'NONE', #5788, #11728 ) ;
#17639=B_SPLINE_CURVE_WITH_KNOTS ( 'NONE', 3,
 ( #9198, #14982, #670, #2708, #11575, #9947 ),
 .UNSPECIFIED., .F., .F.,
 ( 4, 2, 4 ),
 ( 0.000000000000000000, 0.5000000000000000000, 1.000000000000000000 ),
 .UNSPECIFIED. ) ;
#17677=CARTESIAN_POINT ( 'NONE',  ( -9.414213562409999625, -15.31419272936388687, -74.45223986426802298 ) ) ;
#17691=DIRECTION ( 'NONE',  ( -0.7071067811865475727, -0.6644630243886071597, -0.2418447626481610435 ) ) ;
#17722=AXIS2_PLACEMENT_3D ( 'NONE', #2627, #14015, #29203 ) ;
#17749=DIRECTION ( 'NONE',  ( 0.000000000000000000, 0.3420201433259318358, -0.9396926207858125046 ) ) ;
#17759=EDGE_CURVE ( 'NONE', #8329, #13375, #21593, .T. ) ;
#17791=CIRCLE ( 'NONE', #6757, 2.000000000000000000 ) ;
#17812=CARTESIAN_POINT ( 'NONE',  ( -8.000000000000000000, -15.18061163548115466, -76.53197586718597734 ) ) ;
#17828=CARTESIAN_POINT ( 'NONE',  ( 0.000000000000000000, -31.83942647549183746, -80.46693306215520636 ) ) ;
#17837=DIRECTION ( 'NONE',  ( -1.000000000000000000, 0.000000000000000000, 0.000000000000000000 ) ) ;
#17895=ORIENTED_EDGE ( 'NONE', *, *, #3075, .T. ) ;
#17945=CARTESIAN_POINT ( 'NONE',  ( -11.26179938759879740, 26.42151601322855115, -59.26168417594740845 ) ) ;
#17962=ORIENTED_EDGE ( 'NONE', *, *, #25713, .F. ) ;
#17994=CYLINDRICAL_SURFACE ( 'NONE', #21343, 2.000000000000004441 ) ;
#18026=CARTESIAN_POINT ( 'NONE',  ( 7.738200612013472757, -15.86465192213300845, -74.65259062561435144 ) ) ;
#18069=ORIENTED_EDGE ( 'NONE', *, *, #3201, .F. ) ;
#18094=PRESENTATION_STYLE_ASSIGNMENT (( #1284 ) ) ;
#18102=ORIENTED_EDGE ( 'NONE', *, *, #26237, .F. ) ;
#18152=B_SPLINE_CURVE_WITH_KNOTS ( 'NONE', 3,
 ( #21020, #30623, #18495, #4024, #1517, #13775, #28093, #18644, #11574, #3866, #27773, #28242 ),
 .UNSPECIFIED., .F., .F.,
 ( 4, 2, 2, 2, 2, 4 ),
 ( 0.000000000000000000, 0.1250000000000003886, 0.2500000000000007216, 0.5000000000000003331, 0.7500000000000001110, 1.000000000000000000 ),
 .UNSPECIFIED. ) ;
#18183=CARTESIAN_POINT ( 'NONE',  ( -4.000000000000000000, -31.15538618883996946, -82.34631830372681804 ) ) ;
#18198=DIRECTION ( 'NONE',  ( 0.000000000000000000, 0.9396926207858125046, 0.3420201433259318358 ) ) ;
#18204=LINE ( 'NONE', #13655, #29364 ) ;
#18229=ADVANCED_FACE ( 'NONE', ( #19345 ), #2813, .T. ) ;
#18235=CARTESIAN_POINT ( 'NONE',  ( -10.00000000000000000, -13.98526668056139144, -73.96855033896248699 ) ) ;
#18258=CARTESIAN_POINT ( 'NONE',  ( 0.000000000000000000, 22.40709319595134730, -62.85117013414870257 ) ) ;
#18267=VECTOR ( 'NONE', #21553, 1000.000000000000114 ) ;
#18298=VECTOR ( 'NONE', #19696, 1000.000000000000114 ) ;
#18311=DIRECTION ( 'NONE',  ( -1.000000000000000000, 0.000000000000000000, 0.000000000000000000 ) ) ;
#18343=EDGE_CURVE ( 'NONE', #24119, #29525, #17582, .T. ) ;
#18353=ORIENTED_EDGE ( 'NONE', *, *, #30622, .F. ) ;
#18361=AXIS2_PLACEMENT_3D ( 'NONE', #17192, #12164, #23986 ) ;
#18409=CARTESIAN_POINT ( 'NONE',  ( -3.766115772130143036, -0.5867141459235316603, -69.09187603409807821 ) ) ;
#18442=DIRECTION ( 'NONE',  ( 0.000000000000000000, -0.3420201433259318913, 0.9396926207858126157 ) ) ;
#18449=ORIENTED_EDGE ( 'NONE', *, *, #14527, .F. ) ;
#18495=CARTESIAN_POINT ( 'NONE',  ( 0.4344627458603688153, 2.676789689232947467, -67.90405777868647874 ) ) ;
#18513=VERTEX_POINT ( 'NONE', #15409 ) ;
#18514=DIRECTION ( 'NONE',  ( 0.7071067811865467956, 0.6644630243886068266, 0.2418447626481644297 ) ) ;
#18525=EDGE_CURVE ( 'NONE', #22642, #29777, #3293, .T. ) ;
#18533=VERTEX_POINT ( 'NONE', #10543 ) ;
#18555=VECTOR ( 'NONE', #7592, 1000.000000000000114 ) ;
#18573=VERTEX_POINT ( 'NONE', #20138 ) ;
#18624=ORIENTED_EDGE ( 'NONE', *, *, #8753, .F. ) ;
#18634=CARTESIAN_POINT ( 'NONE',  ( -5.414213562369999622, -31.28896728272270877, -80.26658230080884948 ) ) ;
#18644=CARTESIAN_POINT ( 'NONE',  ( 2.731088122681216923, 1.619435980086911586, -68.28890305590695675 ) ) ;
#18663=ORIENTED_EDGE ( 'NONE', *, *, #1377, .T. ) ;
#18685=VECTOR ( 'NONE', #11902, 1000.000000000000114 ) ;
#18714=DIRECTION ( 'NONE',  ( -1.000000000000000000, 0.000000000000000000, 0.000000000000000000 ) ) ;
#18727=EDGE_CURVE ( 'NONE', #15436, #31086, #9889, .T. ) ;
#18765=VERTEX_POINT ( 'NONE', #12400 ) ;
#18783=FACE_OUTER_BOUND ( 'NONE', #13382, .T. ) ;
#18788=LINE ( 'NONE', #24142, #29779 ) ;
#18795=DIRECTION ( 'NONE',  ( 0.7071067811865475727, -0.6644630243886071597, -0.2418447626481610435 ) ) ;
#18796=AXIS2_PLACEMENT_3D ( 'NONE', #29510, #7947, #17691 ) ;
#18820=CARTESIAN_POINT ( 'NONE',  ( 0.000000000000000000, 5.495185456771864096, -69.00660115587162124 ) ) ;
#18822=ORIENTED_EDGE ( 'NONE', *, *, #29259, .F. ) ;
#18851=COLOUR_RGB ( '', 0.66274510, 0.83137255, 0.94901961) ;
#18884=ORIENTED_EDGE ( 'NONE', *, *, #5232, .F. ) ;
#18891=ORIENTED_EDGE ( 'NONE', *, *, #24110, .F. ) ;
#18924=ORIENTED_EDGE ( 'NONE', *, *, #14258, .T. ) ;
#18954=ADVANCED_FACE ( 'NONE', ( #5929 ), #21047, .F. ) ;
#18955=CARTESIAN_POINT ( 'NONE',  ( 12.41421356240000051, 25.87105682045942245, -59.46203493729375822 ) ) ;
#18996=VERTEX_POINT ( 'NONE', #22938 ) ;
#19006=CARTESIAN_POINT ( 'NONE',  ( 6.000000000000000000, -23.85203919881242385, -77.55976184388477179 ) ) ;
#19012=CARTESIAN_POINT ( 'NONE',  ( -4.000000000000000000, -31.83942647549183746, -80.46693306215520636 ) ) ;
#19033=EDGE_LOOP ( 'NONE', ( #5762, #10570, #20233, #17130, #13767, #18663, #22957, #30745, #4032, #9633 ) ) ;
#19034=DIRECTION ( 'NONE',  ( 0.000000000000000000, 0.3420201433259318358, -0.9396926207858125046 ) ) ;
#19062=DIRECTION ( 'NONE',  ( 0.000000000000000000, 0.9396926207858125046, 0.3420201433259318358 ) ) ;
#19071=ORIENTED_EDGE ( 'NONE', *, *, #20716, .F. ) ;
#19090=ORIENTED_EDGE ( 'NONE', *, *, #11820, .F. ) ;
#19092=DIRECTION ( 'NONE',  ( 1.000000000000000000, -0.000000000000000000, 0.000000000000000000 ) ) ;
#19106=EDGE_CURVE ( 'NONE', #18533, #13699, #23878, .T. ) ;
#19137=CARTESIAN_POINT ( 'NONE',  ( -6.000000000000000000, -17.74403716370463968, -75.33663091226621589 ) ) ;
#19144=LINE ( 'NONE', #26390, #11508 ) ;
#19145=DIRECTION ( 'NONE',  ( -1.000000000000000000, 0.000000000000000000, 0.000000000000000000 ) ) ;
#19149=CARTESIAN_POINT ( 'NONE',  ( -6.000000000000000000, -17.74403716370463968, -75.33663091226621589 ) ) ;
#19191=CARTESIAN_POINT ( 'NONE',  ( 4.262644516445695864, -31.82750668785732628, -80.46259461425745485 ) ) ;
#19197=ORIENTED_EDGE ( 'NONE', *, *, #16712, .F. ) ;
#19201=LINE ( 'NONE', #4884, #2442 ) ;
#19218=DIRECTION ( 'NONE',  ( 0.000000000000000000, 0.3420201433259318358, -0.9396926207858125046 ) ) ;
#19220=CARTESIAN_POINT ( 'NONE',  ( 12.41421356240000051, 25.87105682045942245, -59.46203493729375822 ) ) ;
#19223=APPLICATION_CONTEXT ( 'automotive_design' ) ;
#19235=ORIENTED_EDGE ( 'NONE', *, *, #13840, .T. ) ;
#19245=LINE ( 'NONE', #28533, #20702 ) ;
#19268=CYLINDRICAL_SURFACE ( 'NONE', #2573, 2.000000000000002665 ) ;
#19286=LINE ( 'NONE', #7328, #4004 ) ;
#19312=EDGE_CURVE ( 'NONE', #26555, #1709, #16432, .T. ) ;
#19314=EDGE_CURVE ( 'NONE', #2111, #6473, #5200, .T. ) ;
#19329=DIRECTION ( 'NONE',  ( -0.9831920802501790124, -0.1715636151751586680, -0.06244404920691486172 ) ) ;
#19345=FACE_OUTER_BOUND ( 'NONE', #21253, .T. ) ;
#19351=EDGE_CURVE ( 'NONE', #29142, #4930, #9037, .T. ) ;
#19393=DIRECTION ( 'NONE',  ( -1.000000000000000000, 0.000000000000000000, 0.000000000000000000 ) ) ;
#19408=EDGE_LOOP ( 'NONE', ( #26097, #14996, #21541, #13251 ) ) ;
#19483=EDGE_CURVE ( 'NONE', #18533, #20783, #24873, .T. ) ;
#19494=DIRECTION ( 'NONE',  ( 0.000000000000000000, 0.3420201433259318358, -0.9396926207858125046 ) ) ;
#19532=VECTOR ( 'NONE', #3364, 1000.000000000000114 ) ;
#19547=EDGE_LOOP ( 'NONE', ( #1702, #394, #8646, #24729 ) ) ;
#19553=ORIENTED_EDGE ( 'NONE', *, *, #15294, .F. ) ;
#19562=CARTESIAN_POINT ( 'NONE',  ( 1.346291201779999946, -3.434453875705480108, -72.25672407562892374 ) ) ;
#19569=CARTESIAN_POINT ( 'NONE',  ( -13.00000000000000000, 25.22617105830878614, -61.82510970417090590 ) ) ;
#19584=ORIENTED_EDGE ( 'NONE', *, *, #2695, .T. ) ;
#19614=( GEOMETRIC_REPRESENTATION_CONTEXT ( 3 ) GLOBAL_UNCERTAINTY_ASSIGNED_CONTEXT ( ( #24511 ) ) GLOBAL_UNIT_ASSIGNED_CONTEXT ( ( #572, #8230, #13117 ) ) REPRESENTATION_CONTEXT ( 'NONE', 'WORKASPACE' ) );
#19628=ORIENTED_EDGE ( 'NONE', *, *, #21019, .T. ) ;
#19660=ORIENTED_EDGE ( 'NONE', *, *, #26750, .F. ) ;
#19685=CARTESIAN_POINT ( 'NONE',  ( 6.000000000000000000, -29.96004123392021157, -79.78289277550334191 ) ) ;
#19696=DIRECTION ( 'NONE',  ( 0.000000000000000000, 0.3420201433259318358, -0.9396926207858125046 ) ) ;
#19735=AXIS2_PLACEMENT_3D ( 'NONE', #14230, #21468, #9341 ) ;
#19743=ORIENTED_EDGE ( 'NONE', *, *, #5377, .F. ) ;
#19751=AXIS2_PLACEMENT_3D ( 'NONE', #2616, #12208, #19145 ) ;
#19754=VERTEX_POINT ( 'NONE', #15227 ) ;
#19924=CYLINDRICAL_SURFACE ( 'NONE', #18796, 2.000000000000002665 ) ;
#19944=ORIENTED_EDGE ( 'NONE', *, *, #30631, .T. ) ;
#19984=CARTESIAN_POINT ( 'NONE',  ( 3.486379379821376467, -2.190177001292808789, -69.67548878520450728 ) ) ;
#20001=CARTESIAN_POINT ( 'NONE',  ( 13.00000000000000000, 22.06507305262541863, -61.91147751336289673 ) ) ;
#20008=EDGE_LOOP ( 'NONE', ( #16992, #21115, #9903, #6428 ) ) ;
#20025=CARTESIAN_POINT ( 'NONE',  ( 8.000000000050000892, -13.30122639390952877, -75.84793558053411289 ) ) ;
#20026=ADVANCED_FACE ( 'NONE', ( #12212 ), #21824, .F. ) ;
#20027=DIRECTION ( 'NONE',  ( 0.000000000000000000, 0.3420201433259318358, -0.9396926207858125046 ) ) ;
#20029=AXIS2_PLACEMENT_3D ( 'NONE', #21216, #16489, #4538 ) ;
#20134=DIRECTION ( 'NONE',  ( 0.000000000000000000, -0.3420201433259318913, 0.9396926207858126157 ) ) ;
#20138=CARTESIAN_POINT ( 'NONE',  ( 6.000000000000000000, -17.05999687705277879, -77.21601615383784178 ) ) ;
#20178=PLANE ( 'NONE',  #14031 ) ;
#20206=SURFACE_STYLE_USAGE ( .BOTH. , #12969 ) ;
#20208=ORIENTED_EDGE ( 'NONE', *, *, #13481, .T. ) ;
#20233=ORIENTED_EDGE ( 'NONE', *, *, #7472, .T. ) ;
#20289=DIRECTION ( 'NONE',  ( 1.000000000000000000, 0.000000000000000000, 0.000000000000000000 ) ) ;
#20326=ADVANCED_FACE ( 'NONE', ( #2291 ), #30764, .T. ) ;
#20343=AXIS2_PLACEMENT_3D ( 'NONE', #24295, #29314, #703 ) ;
#20356=CIRCLE ( 'NONE', #24879, 2.000000000000000000 ) ;
#20360=ADVANCED_FACE ( 'NONE', ( #9193 ), #19268, .T. ) ;
#20427=ORIENTED_EDGE ( 'NONE', *, *, #12699, .F. ) ;
#20508=ORIENTED_EDGE ( 'NONE', *, *, #5387, .F. ) ;
#20542=ADVANCED_FACE ( 'NONE', ( #31015 ), #28794, .T. ) ;
#20549=ORIENTED_EDGE ( 'NONE', *, *, #4532, .T. ) ;
#20645=CARTESIAN_POINT ( 'NONE',  ( 5.414213562369999622, -31.28896728272270877, -80.26658230080884948 ) ) ;
#20647=CARTESIAN_POINT ( 'NONE',  ( -10.00000000000000000, 22.06507305262541863, -61.91147751336289673 ) ) ;
#20659=DIRECTION ( 'NONE',  ( 0.000000000000000000, 0.9396926207858125046, 0.3420201433259318358 ) ) ;
#20672=DIRECTION ( 'NONE',  ( -1.000000000000000000, 0.000000000000000000, 0.000000000000000000 ) ) ;
#20678=AXIS2_PLACEMENT_3D ( 'NONE', #151, #11790, #14770 ) ;
#20695=LINE ( 'NONE', #27304, #7733 ) ;
#20696=ORIENTED_EDGE ( 'NONE', *, *, #20844, .T. ) ;
#20699=VECTOR ( 'NONE', #13925, 1000.000000000000114 ) ;
#20702=VECTOR ( 'NONE', #19092, 1000.000000000000000 ) ;
#20709=ORIENTED_EDGE ( 'NONE', *, *, #15160, .T. ) ;
#20715=CIRCLE ( 'NONE', #29262, 3.750000000000000000 ) ;
#20716=EDGE_CURVE ( 'NONE', #8641, #3121, #13568, .T. ) ;
#20773=CARTESIAN_POINT ( 'NONE',  ( -2.783363191001295700, -3.225935323956106604, -70.05247398454777397 ) ) ;
#20780=ORIENTED_EDGE ( 'NONE', *, *, #22973, .F. ) ;
#20782=ORIENTED_EDGE ( 'NONE', *, *, #23903, .F. ) ;
#20783=VERTEX_POINT ( 'NONE', #12292 ) ;
#20793=EDGE_CURVE ( 'NONE', #22642, #2258, #3495, .T. ) ;
#20799=ORIENTED_EDGE ( 'NONE', *, *, #15979, .T. ) ;
#20824=ORIENTED_EDGE ( 'NONE', *, *, #20793, .T. ) ;
#20844=EDGE_CURVE ( 'NONE', #29055, #8641, #10977, .T. ) ;
#20887=CARTESIAN_POINT ( 'NONE',  ( 6.992762038593867580, -16.10185592147890077, -74.73892582082525848 ) ) ;
#20889=AXIS2_PLACEMENT_3D ( 'NONE', #8830, #13718, #20958 ) ;
#20891=FACE_OUTER_BOUND ( 'NONE', #22785, .T. ) ;
#20934=ORIENTED_EDGE ( 'NONE', *, *, #15759, .T. ) ;
#20958=DIRECTION ( 'NONE',  ( -1.000000000000000000, 0.000000000000000000, 0.000000000000000000 ) ) ;
#20965=PLANE ( 'NONE',  #13233 ) ;
#20978=DIRECTION ( 'NONE',  ( 0.000000000000000000, -0.3420201433259318358, 0.9396926207858125046 ) ) ;
#20990=VECTOR ( 'NONE', #25644, 1000.000000000000000 ) ;
#21003=DIRECTION ( 'NONE',  ( 0.9831920802501790124, 0.1715636151751586680, 0.06244404920691486172 ) ) ;
#21019=EDGE_CURVE ( 'NONE', #29115, #28085, #2201, .T. ) ;
#21020=CARTESIAN_POINT ( 'NONE',  ( 2.664535259099999805E-15, 2.694277338339796213, -67.89769279494430521 ) ) ;
#21022=EDGE_CURVE ( 'NONE', #14059, #2111, #2356, .T. ) ;
#21027=ADVANCED_FACE ( 'NONE', ( #7671 ), #28624, .T. ) ;
#21030=B_SPLINE_CURVE_WITH_KNOTS ( 'NONE', 3,
 ( #9118, #28319, #19191, #21406, #9272, #21244, #6606, #23770 ),
 .UNSPECIFIED., .F., .F.,
 ( 4, 2, 2, 4 ),
 ( 0.000000000000000000, 0.2500000000000000555, 0.5000000000000001110, 1.000000000000000000 ),
 .UNSPECIFIED. ) ;
#21047=CYLINDRICAL_SURFACE ( 'NONE', #27226, 2.000000000000003553 ) ;
#21058=EDGE_CURVE ( 'NONE', #11115, #10219, #7109, .T. ) ;
#21079=ORIENTED_EDGE ( 'NONE', *, *, #28189, .T. ) ;
#21083=CIRCLE ( 'NONE', #4503, 2.000000000000000000 ) ;
#21092=CARTESIAN_POINT ( 'NONE',  ( -2.128136350289183021, -3.759461034538412516, -70.24666146241560227 ) ) ;
#21115=ORIENTED_EDGE ( 'NONE', *, *, #15759, .F. ) ;
#21119=LINE ( 'NONE', #25691, #3628 ) ;
#21214=ORIENTED_EDGE ( 'NONE', *, *, #16820, .F. ) ;
#21216=CARTESIAN_POINT ( 'NONE',  ( -11.00000000000000000, 25.22617105830878614, -61.82510970417090590 ) ) ;
#21244=CARTESIAN_POINT ( 'NONE',  ( 5.007332623075492428, -31.60226355569895773, -80.38061281867886976 ) ) ;
#21251=EDGE_LOOP ( 'NONE', ( #3280, #7769, #29936, #2827 ) ) ;
#21253=EDGE_LOOP ( 'NONE', ( #13823, #1274, #19071, #2027 ) ) ;
#21308=DIRECTION ( 'NONE',  ( 0.000000000000000000, 0.3420201433259318913, -0.9396926207858126157 ) ) ;
#21311=CARTESIAN_POINT ( 'NONE',  ( -2.220446049249999755E-16, -0.1455297029551360921, -71.05965357398815740 ) ) ;
#21317=FACE_OUTER_BOUND ( 'NONE', #28684, .T. ) ;
#21340=VECTOR ( 'NONE', #21985, 1000.000000000000000 ) ;
#21343=AXIS2_PLACEMENT_3D ( 'NONE', #30129, #24942, #25423 ) ;
#21376=ORIENTED_EDGE ( 'NONE', *, *, #18525, .T. ) ;
#21406=CARTESIAN_POINT ( 'NONE',  ( 4.517774681172858742, -31.77982753731929577, -80.44524082266653409 ) ) ;
#21446=EDGE_LOOP ( 'NONE', ( #7360, #21886, #894, #31083 ) ) ;
#21461=ORIENTED_EDGE ( 'NONE', *, *, #30801, .T. ) ;
#21468=DIRECTION ( 'NONE',  ( 0.000000000000000000, -0.3420201433259318913, 0.9396926207858126157 ) ) ;
#21541=ORIENTED_EDGE ( 'NONE', *, *, #14555, .T. ) ;
#21551=ADVANCED_FACE ( 'NONE', ( #1039 ), #24949, .T. ) ;
#21553=DIRECTION ( 'NONE',  ( 0.000000000000000000, 0.9396926207858125046, 0.3420201433259318358 ) ) ;
#21579=ADVANCED_FACE ( 'NONE', ( #10628 ), #19924, .T. ) ;
#21591=CARTESIAN_POINT ( 'NONE',  ( 12.59933368536904297, 25.69710080669531038, -59.52534974837554671 ) ) ;
#21593=LINE ( 'NONE', #1930, #17244 ) ;
#21595=CARTESIAN_POINT ( 'NONE',  ( -9.414213562409999625, -14.63015244271202420, -76.33162510583964888 ) ) ;
#21616=CARTESIAN_POINT ( 'NONE',  ( 4.440892098500000496E-16, -0.1455297029551360921, -71.05965357398815740 ) ) ;
#21653=DIRECTION ( 'NONE',  ( -1.000000000000000000, 0.000000000000000000, 0.000000000000000000 ) ) ;
#21684=DIRECTION ( 'NONE',  ( 0.000000000000000000, 0.3420201433259318358, -0.9396926207858125046 ) ) ;
#21701=DIRECTION ( 'NONE',  ( 1.000000000000000000, -0.000000000000000000, 0.000000000000000000 ) ) ;
#21800=EDGE_CURVE ( 'NONE', #2111, #1677, #2891, .T. ) ;
#21818=CARTESIAN_POINT ( 'NONE',  ( -4.000000000000000000, -31.83942647549183746, -80.46693306215520636 ) ) ;
#21824=PLANE ( 'NONE',  #5571 ) ;
#21848=CARTESIAN_POINT ( 'NONE',  ( 3.686970300939999667, 0.4978338539504151838, -70.82548838946271985 ) ) ;
#21886=ORIENTED_EDGE ( 'NONE', *, *, #14447, .T. ) ;
#21897=EDGE_LOOP ( 'NONE', ( #4886, #30560, #23971, #3463, #31098, #30599, #11185, #6984, #22635, #21461 ) ) ;
#21907=EDGE_CURVE ( 'NONE', #17565, #3121, #10774, .T. ) ;
#21919=VERTEX_POINT ( 'NONE', #29474 ) ;
#21921=EDGE_LOOP ( 'NONE', ( #27860, #3472, #7426, #26506, #24757, #3124, #12375, #29963, #18102, #14567 ) ) ;
#21922=VERTEX_POINT ( 'NONE', #17812 ) ;
#21956=ORIENTED_EDGE ( 'NONE', *, *, #29890, .F. ) ;
#21985=DIRECTION ( 'NONE',  ( 1.000000000000000000, -0.000000000000000000, 0.000000000000000000 ) ) ;
#21989=DIRECTION ( 'NONE',  ( 0.000000000000000000, -0.3420201433259318358, 0.9396926207858125046 ) ) ;
#21999=PLANE ( 'NONE',  #29571 ) ;
#22014=DIRECTION ( 'NONE',  ( 0.000000000000000000, 0.3420201433259318913, -0.9396926207858126157 ) ) ;
#22020=DIRECTION ( 'NONE',  ( -0.7071067811865467956, 0.6644630243886068266, 0.2418447626481644297 ) ) ;
#22034=ORIENTED_EDGE ( 'NONE', *, *, #22523, .T. ) ;
#22042=DIRECTION ( 'NONE',  ( 0.000000000000000000, -0.9396926207858125046, -0.3420201433259318358 ) ) ;
#22055=CARTESIAN_POINT ( 'NONE',  ( 9.414213562409999625, -15.31419272936388687, -74.45223986426802298 ) ) ;
#22056=CARTESIAN_POINT ( 'NONE',  ( 5.414213562369999622, -31.28896728272270877, -80.26658230080884948 ) ) ;
#22064=CARTESIAN_POINT ( 'NONE',  ( 11.00000000000000000, 27.10555629988041204, -61.14106941751904856 ) ) ;
#22073=ORIENTED_EDGE ( 'NONE', *, *, #15387, .F. ) ;
#22074=VECTOR ( 'NONE', #6007, 1000.000000000000114 ) ;
#22084=CARTESIAN_POINT ( 'NONE',  ( -8.000000000000000000, -15.86465192213301556, -74.65259062561435144 ) ) ;
#22092=CARTESIAN_POINT ( 'NONE',  ( 0.000000000000000000, -15.18061163548115466, -76.53197586718597734 ) ) ;
#22101=ADVANCED_FACE ( 'NONE', ( #15934 ), #27729, .F. ) ;
#22118=VERTEX_POINT ( 'NONE', #6337 ) ;
#22131=CIRCLE ( 'NONE', #30670, 2.000000000000000000 ) ;
#22167=CARTESIAN_POINT ( 'NONE',  ( 6.000000000000000000, -23.16799891216055940, -79.43914708545641190 ) ) ;
#22170=LINE ( 'NONE', #26432, #8728 ) ;
#22199=CARTESIAN_POINT ( 'NONE',  ( 8.523495768347459034, -15.81573655486863750, -74.63478688793190940 ) ) ;
#22208=ORIENTED_EDGE ( 'NONE', *, *, #22523, .F. ) ;
#22213=VERTEX_POINT ( 'NONE', #22479 ) ;
#22244=EDGE_LOOP ( 'NONE', ( #10498, #13104, #16838, #8278, #27588, #22208 ) ) ;
#22247=DIRECTION ( 'NONE',  ( 0.000000000000000000, -0.9396926207858125046, -0.3420201433259318358 ) ) ;
#22276=CARTESIAN_POINT ( 'NONE',  ( -5.600170770410507259, -31.11415510469601031, -80.20295587141983162 ) ) ;
#22334=EDGE_CURVE ( 'NONE', #9128, #21922, #1855, .T. ) ;
#22348=VECTOR ( 'NONE', #23498, 1000.000000000000000 ) ;
#22358=B_SPLINE_CURVE_WITH_KNOTS ( 'NONE', 3,
 ( #23768, #18409, #25818, #1894, #16514, #27853, #20773, #21092, #2209, #6302 ),
 .UNSPECIFIED., .F., .F.,
 ( 4, 2, 2, 2, 4 ),
 ( 0.000000000000000000, 0.2499999999999998890, 0.4999999999999997780, 0.7499999999999998890, 1.000000000000000000 ),
 .UNSPECIFIED. ) ;
#22370=EDGE_CURVE ( 'NONE', #7467, #26555, #18204, .T. ) ;
#22399=CARTESIAN_POINT ( 'NONE',  ( -6.585786437629999490, -16.41511111490214603, -74.85294138696069410 ) ) ;
#22423=PLANE ( 'NONE',  #26232 ) ;
#22479=CARTESIAN_POINT ( 'NONE',  ( -12.41421356240000051, 25.87105682045942245, -59.46203493729375822 ) ) ;
#22494=ORIENTED_EDGE ( 'NONE', *, *, #19314, .T. ) ;
#22518=CARTESIAN_POINT ( 'NONE',  ( -9.747572777117802900, -14.93176075901369515, -74.31304601042864988 ) ) ;
#22522=ADVANCED_FACE ( 'NONE', ( #28902 ), #23890, .T. ) ;
#22523=EDGE_CURVE ( 'NONE', #23530, #29115, #24340, .T. ) ;
#22526=ORIENTED_EDGE ( 'NONE', *, *, #21058, .F. ) ;
#22538=CARTESIAN_POINT ( 'NONE',  ( -3.454061855166487671, 0.6016891855815794665, -68.65933259512706854 ) ) ;
#22580=FILL_AREA_STYLE ('',( #5276 ) ) ;
#22597=DIRECTION ( 'NONE',  ( -1.000000000000000000, 0.000000000000000000, 0.000000000000000000 ) ) ;
#22635=ORIENTED_EDGE ( 'NONE', *, *, #11820, .T. ) ;
#22642=VERTEX_POINT ( 'NONE', #18955 ) ;
#22648=DIRECTION ( 'NONE',  ( -0.7071067811780481493, 0.6644630243965948813, 0.2418447626510653869 ) ) ;
#22682=CARTESIAN_POINT ( 'NONE',  ( -3.686970300939999667, -0.1862064327014488485, -68.94610314789107974 ) ) ;
#22686=FACE_OUTER_BOUND ( 'NONE', #30432, .T. ) ;
#22785=EDGE_LOOP ( 'NONE', ( #1080, #16374, #26897, #17962 ) ) ;
#22870=VECTOR ( 'NONE', #10258, 1000.000000000000114 ) ;
#22938=CARTESIAN_POINT ( 'NONE',  ( 6.585786437629999490, -15.73107082825028336, -76.73232662853232000 ) ) ;
#22957=ORIENTED_EDGE ( 'NONE', *, *, #1176, .T. ) ;
#22973=EDGE_CURVE ( 'NONE', #2672, #29525, #29597, .T. ) ;
#22985=ORIENTED_EDGE ( 'NONE', *, *, #21022, .T. ) ;
#22994=( LENGTH_UNIT ( ) NAMED_UNIT ( * ) SI_UNIT ( .MILLI., .METRE. ) );
#23114=ORIENTED_EDGE ( 'NONE', *, *, #19312, .T. ) ;
#23133=FACE_OUTER_BOUND ( 'NONE', #25828, .T. ) ;
#23154=ORIENTED_EDGE ( 'NONE', *, *, #28989, .T. ) ;
#23178=DIRECTION ( 'NONE',  ( 0.000000000000000000, -0.3420201433259318913, 0.9396926207858126157 ) ) ;
#23180=ORIENTED_EDGE ( 'NONE', *, *, #5387, .T. ) ;
#23194=VERTEX_POINT ( 'NONE', #3464 ) ;
#23218=CARTESIAN_POINT ( 'NONE',  ( 13.00000000000000000, 25.22617105830878614, -61.82510970417090590 ) ) ;
#23229=CARTESIAN_POINT ( 'NONE',  ( 3.686970300939999667, -0.1862064327014488485, -68.94610314789109395 ) ) ;
#23245=EDGE_LOOP ( 'NONE', ( #11092, #27323, #21079, #27359 ) ) ;
#23291=EDGE_CURVE ( 'NONE', #10428, #18996, #8332, .T. ) ;
#23296=CARTESIAN_POINT ( 'NONE',  ( -6.000000000000000000, -17.40201702037870746, -76.27632353305202173 ) ) ;
#23342=EDGE_CURVE ( 'NONE', #15436, #29055, #21030, .T. ) ;
#23382=EDGE_CURVE ( 'NONE', #10428, #1677, #13897, .T. ) ;
#23468=ORIENTED_EDGE ( 'NONE', *, *, #23759, .T. ) ;
#23482=FACE_OUTER_BOUND ( 'NONE', #6838, .T. ) ;
#23497=CARTESIAN_POINT ( 'NONE',  ( 5.414213562369999622, -31.28896728272270877, -80.26658230080884948 ) ) ;
#23498=DIRECTION ( 'NONE',  ( 1.000000000000000000, -0.000000000000000000, 0.000000000000000000 ) ) ;
#23530=VERTEX_POINT ( 'NONE', #4360 ) ;
#23555=AXIS2_PLACEMENT_3D ( 'NONE', #14654, #12431, #26755 ) ;
#23613=CARTESIAN_POINT ( 'NONE',  ( -12.41421356240000051, 26.55509710711128335, -61.34142017886538412 ) ) ;
#23677=AXIS2_PLACEMENT_3D ( 'NONE', #1980, #26356, #31074 ) ;
#23691=ORIENTED_EDGE ( 'NONE', *, *, #16182, .T. ) ;
#23700=ORIENTED_EDGE ( 'NONE', *, *, #29385, .T. ) ;
#23751=CARTESIAN_POINT ( 'NONE',  ( -2.220446049249999755E-16, -0.1455297029551360921, -71.05965357398815740 ) ) ;
#23759=EDGE_CURVE ( 'NONE', #25602, #28085, #5288, .T. ) ;
#23768=CARTESIAN_POINT ( 'NONE',  ( -3.686970300939999667, -0.1862064327014488485, -68.94610314789107974 ) ) ;
#23770=CARTESIAN_POINT ( 'NONE',  ( 5.414213562369999622, -31.28896728272270877, -80.26658230080884948 ) ) ;
#23812=ORIENTED_EDGE ( 'NONE', *, *, #446, .F. ) ;
#23835=CYLINDRICAL_SURFACE ( 'NONE', #19735, 2.000000000000000000 ) ;
#23867=AXIS2_PLACEMENT_3D ( 'NONE', #8249, #6211, #25103 ) ;
#23878=LINE ( 'NONE', #2468, #18685 ) ;
#23883=EDGE_CURVE ( 'NONE', #16796, #8103, #29596, .T. ) ;
#23890=CYLINDRICAL_SURFACE ( 'NONE', #3744, 2.000000000000003553 ) ;
#23903=EDGE_CURVE ( 'NONE', #29525, #1709, #20695, .T. ) ;
#23928=CARTESIAN_POINT ( 'NONE',  ( 6.252427222934309192, -16.79754308524862694, -74.99213524079873139 ) ) ;
#23938=DIRECTION ( 'NONE',  ( -1.000000000000000000, 0.000000000000000000, 0.000000000000000000 ) ) ;
#23971=ORIENTED_EDGE ( 'NONE', *, *, #24110, .T. ) ;
#23976=EDGE_LOOP ( 'NONE', ( #14983, #1247, #18624, #24503 ) ) ;
#23979=EDGE_CURVE ( 'NONE', #7544, #13699, #15651, .T. ) ;
#23986=DIRECTION ( 'NONE',  ( -1.000000000000000000, 0.000000000000000000, 0.000000000000000000 ) ) ;
#23990=ORIENTED_EDGE ( 'NONE', *, *, #17346, .F. ) ;
#24001=CARTESIAN_POINT ( 'NONE',  ( -11.00000000000000000, 25.22617105830878614, -61.82510970417090590 ) ) ;
#24013=LINE ( 'NONE', #26667, #5368 ) ;
#24037=AXIS2_PLACEMENT_3D ( 'NONE', #14536, #2569, #24130 ) ;
#24110=EDGE_CURVE ( 'NONE', #29777, #24119, #28851, .T. ) ;
#24119=VERTEX_POINT ( 'NONE', #23218 ) ;
#24128=CARTESIAN_POINT ( 'NONE',  ( 4.000000000000000000, -29.27600094726834712, -81.66227801707495360 ) ) ;
#24130=DIRECTION ( 'NONE',  ( -0.7071067811865467956, 0.6644630243886068266, 0.2418447626481644297 ) ) ;
#24142=CARTESIAN_POINT ( 'NONE',  ( 10.00000000000000000, -13.98526668056139144, -73.96855033896248699 ) ) ;
#24144=CARTESIAN_POINT ( 'NONE',  ( 10.00000000000000000, -13.98526668056139144, -73.96855033896248699 ) ) ;
#24147=ADVANCED_FACE ( 'NONE', ( #21317 ), #6529, .T. ) ;
#24164=UNCERTAINTY_MEASURE_WITH_UNIT (LENGTH_MEASURE( 1.000000000000000082E-05 ), #22994, 'distance_accuracy_value', 'NONE');
#24195=EDGE_LOOP ( 'NONE', ( #8457, #15358, #21956, #2368 ) ) ;
#24232=ORIENTED_EDGE ( 'NONE', *, *, #446, .T. ) ;
#24239=AXIS2_PLACEMENT_3D ( 'NONE', #20025, #12166, #29465 ) ;
#24263=DIRECTION ( 'NONE',  ( 0.000000000000000000, 0.9396926207858125046, 0.3420201433259318358 ) ) ;
#24268=VERTEX_POINT ( 'NONE', #24144 ) ;
#24284=AXIS2_PLACEMENT_3D ( 'NONE', #12405, #5018, #22020 ) ;
#24295=CARTESIAN_POINT ( 'NONE',  ( 4.000000000000000000, -29.27600094726834712, -81.66227801707495360 ) ) ;
#24305=CARTESIAN_POINT ( 'NONE',  ( -3.686970300939999667, 0.4978338539504151838, -70.82548838946271985 ) ) ;
#24312=FACE_OUTER_BOUND ( 'NONE', #9713, .T. ) ;
#24329=AXIS2_PLACEMENT_3D ( 'NONE', #25151, #3277, #25310 ) ;
#24340=LINE ( 'NONE', #12373, #21340 ) ;
#24359=DIRECTION ( 'NONE',  ( 0.000000000000000000, -0.3420201433259318913, 0.9396926207858126157 ) ) ;
#24383=EDGE_LOOP ( 'NONE', ( #20782, #20780, #23700, #23114 ) ) ;
#24402=CARTESIAN_POINT ( 'NONE',  ( 12.41421356240000051, 26.55509710711128335, -61.34142017886538412 ) ) ;
#24413=DIRECTION ( 'NONE',  ( 1.000000000000000000, -0.000000000000000000, 0.000000000000000000 ) ) ;
#24497=EDGE_CURVE ( 'NONE', #29115, #24684, #28354, .T. ) ;
#24503=ORIENTED_EDGE ( 'NONE', *, *, #23291, .F. ) ;
#24511=UNCERTAINTY_MEASURE_WITH_UNIT (LENGTH_MEASURE( 1.000000000000000082E-05 ), #572, 'distance_accuracy_value', 'NONE');
#24583=ORIENTED_EDGE ( 'NONE', *, *, #21800, .F. ) ;
#24585=VECTOR ( 'NONE', #14733, 1000.000000000000114 ) ;
#24619=VERTEX_POINT ( 'NONE', #21595 ) ;
#24622=PRODUCT_DEFINITION ( 'UNKNOWN', '', #5308, #11588 ) ;
#24627=DIRECTION ( 'NONE',  ( 0.000000000000000000, -0.3420201433259318913, 0.9396926207858126157 ) ) ;
#24651=DIRECTION ( 'NONE',  ( 0.000000000000000000, -0.3420201433259318913, 0.9396926207858126157 ) ) ;
#24684=VERTEX_POINT ( 'NONE', #44 ) ;
#24707=CARTESIAN_POINT ( 'NONE',  ( 2.125375073177956597, -3.761816432237487628, -70.24751875706795090 ) ) ;
#24729=ORIENTED_EDGE ( 'NONE', *, *, #17346, .T. ) ;
#24749=CARTESIAN_POINT ( 'NONE',  ( -6.000000000000000000, -29.61802109059427934, -80.72258539628914775 ) ) ;
#24757=ORIENTED_EDGE ( 'NONE', *, *, #3020, .F. ) ;
#24784=VERTEX_POINT ( 'NONE', #3456 ) ;
#24871=CARTESIAN_POINT ( 'NONE',  ( -2.220446049249999755E-16, -0.1455297029551360921, -71.05965357398815740 ) ) ;
#24873=LINE ( 'NONE', #1104, #16176 ) ;
#24879=AXIS2_PLACEMENT_3D ( 'NONE', #1336, #24627, #17837 ) ;
#24932=FACE_OUTER_BOUND ( 'NONE', #14100, .T. ) ;
#24942=DIRECTION ( 'NONE',  ( 0.000000000000000000, 0.3420201433259318913, -0.9396926207858126157 ) ) ;
#24949=PLANE ( 'NONE',  #1210 ) ;
#24978=LINE ( 'NONE', #29850, #8984 ) ;
#24983=DIRECTION ( 'NONE',  ( 0.000000000000000000, -0.9396926207858125046, -0.3420201433259318358 ) ) ;
#24991=ORIENTED_EDGE ( 'NONE', *, *, #23342, .F. ) ;
#25018=FACE_OUTER_BOUND ( 'NONE', #4356, .T. ) ;
#25057=DIRECTION ( 'NONE',  ( 0.000000000000000000, 0.3420201433259318913, -0.9396926207858126157 ) ) ;
#25103=DIRECTION ( 'NONE',  ( 0.7071067811865475727, 0.6644630243886071597, 0.2418447626481610435 ) ) ;
#25106=ORIENTED_EDGE ( 'NONE', *, *, #29259, .T. ) ;
#25132=MECHANICAL_DESIGN_GEOMETRIC_PRESENTATION_REPRESENTATION('',(#9047),#19614);
#25151=CARTESIAN_POINT ( 'NONE',  ( -4.000000000000000000, -29.27600094726834712, -81.66227801707495360 ) ) ;
#25166=CARTESIAN_POINT ( 'NONE',  ( 12.00723796141030775, 26.18431201388056095, -59.34801937115905446 ) ) ;
#25233=ORIENTED_EDGE ( 'NONE', *, *, #20793, .F. ) ;
#25253=VECTOR ( 'NONE', #19218, 1000.000000000000114 ) ;
#25292=CARTESIAN_POINT ( 'NONE',  ( 1.755400582548710009, -3.970618665040213546, -70.32351655465652129 ) ) ;
#25296=DIRECTION ( 'NONE',  ( -1.000000000000000000, 0.000000000000000000, 0.000000000000000000 ) ) ;
#25310=DIRECTION ( 'NONE',  ( -1.000000000000000000, 0.000000000000000000, 0.000000000000000000 ) ) ;
#25325=CARTESIAN_POINT ( 'NONE',  ( 12.22909344072123439, 26.04501283290617764, -59.39872012669144397 ) ) ;
#25392=ORIENTED_EDGE ( 'NONE', *, *, #19351, .F. ) ;
#25394=CARTESIAN_POINT ( 'NONE',  ( -3.686970300939999667, 0.4978338539504151838, -70.82548838946271985 ) ) ;
#25423=DIRECTION ( 'NONE',  ( 0.7071067811865469066, -0.6644630243886066046, -0.2418447626481643187 ) ) ;
#25428=CYLINDRICAL_SURFACE ( 'NONE', #23867, 2.000000000000002665 ) ;
#25580=CARTESIAN_POINT ( 'NONE',  ( -13.00000000000000000, 25.22617105830878614, -61.82510970417090590 ) ) ;
#25602=VERTEX_POINT ( 'NONE', #26619 ) ;
#25624=AXIS2_PLACEMENT_3D ( 'NONE', #17073, #29029, #2148 ) ;
#25644=DIRECTION ( 'NONE',  ( -1.000000000000000000, 0.000000000000000000, 0.000000000000000000 ) ) ;
#25686=CARTESIAN_POINT ( 'NONE',  ( -12.00723796003150845, 26.18431201457259050, -59.34801937090718837 ) ) ;
#25690=PLANE ( 'NONE',  #20889 ) ;
#25691=CARTESIAN_POINT ( 'NONE',  ( -13.00000000000000000, 23.13259184047820582, -60.45875467758818189 ) ) ;
#25703=ORIENTED_EDGE ( 'NONE', *, *, #16999, .F. ) ;
#25709=LINE ( 'NONE', #13900, #5740 ) ;
#25713=EDGE_CURVE ( 'NONE', #29142, #3795, #14109, .T. ) ;
#25755=ORIENTED_EDGE ( 'NONE', *, *, #3020, .T. ) ;
#25806=EDGE_CURVE ( 'NONE', #13375, #21919, #28316, .T. ) ;
#25818=CARTESIAN_POINT ( 'NONE',  ( -3.770605797612482490, -1.000149664079264422, -69.24235425649531805 ) ) ;
#25828=EDGE_LOOP ( 'NONE', ( #4062, #22034, #19628, #3202 ) ) ;
#25829=VERTEX_POINT ( 'NONE', #13533 ) ;
#25956=EDGE_CURVE ( 'NONE', #27093, #23530, #22358, .T. ) ;
#26031=VERTEX_POINT ( 'NONE', #28631 ) ;
#26033=EDGE_CURVE ( 'NONE', #1709, #8147, #22170, .T. ) ;
#26035=CARTESIAN_POINT ( 'NONE',  ( 0.000000000000000000, 5.495185456771864096, -69.00660115587162124 ) ) ;
#26097=ORIENTED_EDGE ( 'NONE', *, *, #18727, .F. ) ;
#26114=DIRECTION ( 'NONE',  ( 0.000000000000000000, 0.3420201433259318358, -0.9396926207858125046 ) ) ;
#26150=LINE ( 'NONE', #28798, #3783 ) ;
#26205=CARTESIAN_POINT ( 'NONE',  ( -6.000000000000000000, -16.80434454291883029, -74.99461076894029077 ) ) ;
#26232=AXIS2_PLACEMENT_3D ( 'NONE', #3674, #27438, #6035 ) ;
#26237=EDGE_CURVE ( 'NONE', #21919, #8607, #1392, .T. ) ;
#26244=VECTOR ( 'NONE', #17256, 1000.000000000000114 ) ;
#26304=CARTESIAN_POINT ( 'NONE',  ( 13.00000000000000178, 24.78814172431745533, -59.85618379852729731 ) ) ;
#26331=AXIS2_PLACEMENT_3D ( 'NONE', #3649, #23178, #15311 ) ;
#26356=DIRECTION ( 'NONE',  ( 0.000000000000000000, 0.9396926207858126157, 0.3420201433259318913 ) ) ;
#26390=CARTESIAN_POINT ( 'NONE',  ( -1.346291201779999946, -3.434453875705480108, -72.25672407562892374 ) ) ;
#26395=CARTESIAN_POINT ( 'NONE',  ( -6.585786437629999490, -16.41511111490214603, -74.85294138696069410 ) ) ;
#26398=ORIENTED_EDGE ( 'NONE', *, *, #13481, .F. ) ;
#26432=CARTESIAN_POINT ( 'NONE',  ( 10.00000000000000000, 4.552933401020911042, -69.34955285734142194 ) ) ;
#26478=CARTESIAN_POINT ( 'NONE',  ( 13.00000000000000000, 24.54213077165692525, -59.94572446259928711 ) ) ;
#26506=ORIENTED_EDGE ( 'NONE', *, *, #21907, .F. ) ;
#26536=LINE ( 'NONE', #21818, #24585 ) ;
#26555=VERTEX_POINT ( 'NONE', #1199 ) ;
#26560=DIRECTION ( 'NONE',  ( 0.000000000000000000, 0.9396926207858125046, 0.3420201433259318358 ) ) ;
#26563=FACE_OUTER_BOUND ( 'NONE', #665, .T. ) ;
#26619=CARTESIAN_POINT ( 'NONE',  ( -1.346291201189999898, -3.434453875705480108, -72.25672407562892374 ) ) ;
#26620=VECTOR ( 'NONE', #10381, 1000.000000000000114 ) ;
#26640=DIRECTION ( 'NONE',  ( 0.000000000000000000, 0.3420201433259318358, -0.9396926207858125046 ) ) ;
#26667=CARTESIAN_POINT ( 'NONE',  ( -6.000000000000000000, -16.12030425626696939, -76.87399601051191667 ) ) ;
#26750=EDGE_CURVE ( 'NONE', #22118, #9001, #18152, .T. ) ;
#26755=DIRECTION ( 'NONE',  ( 0.000000000000000000, -0.9396926207858125046, -0.3420201433259318358 ) ) ;
#26759=CARTESIAN_POINT ( 'NONE',  ( 2.787054272977523173, -3.222358495660834876, -70.05117212551519401 ) ) ;
#26793=LINE ( 'NONE', #22084, #7416 ) ;
#26823=CARTESIAN_POINT ( 'NONE',  ( 8.000000000000000000, -15.18061163548115466, -76.53197586718597734 ) ) ;
#26860=ORIENTED_EDGE ( 'NONE', *, *, #14527, .T. ) ;
#26892=VECTOR ( 'NONE', #13390, 1000.000000000000000 ) ;
#26897=ORIENTED_EDGE ( 'NONE', *, *, #14555, .F. ) ;
#26919=CARTESIAN_POINT ( 'NONE',  ( 3.629192601380414551, -1.807102915225842432, -69.53606122035726855 ) ) ;
#26936=ORIENTED_EDGE ( 'NONE', *, *, #16820, .T. ) ;
#27068=CARTESIAN_POINT ( 'NONE',  ( -7.737355262860049265, -15.87657168464556534, -74.65692906436845533 ) ) ;
#27071=EDGE_CURVE ( 'NONE', #11066, #1347, #2211, .T. ) ;
#27093=VERTEX_POINT ( 'NONE', #1321 ) ;
#27111=LINE ( 'NONE', #20647, #17313 ) ;
#27139=DIRECTION ( 'NONE',  ( 0.000000000000000000, 0.3420201433259318913, -0.9396926207858126157 ) ) ;
#27147=CARTESIAN_POINT ( 'NONE',  ( -8.000000000000000000, -17.05999687705277879, -77.21601615383784178 ) ) ;
#27226=AXIS2_PLACEMENT_3D ( 'NONE', #10822, #8436, #3570 ) ;
#27245=AXIS2_PLACEMENT_3D ( 'NONE', #8393, #30452, #1181 ) ;
#27261=DIRECTION ( 'NONE',  ( 0.000000000000000000, 0.9396926207858125046, 0.3420201433259318358 ) ) ;
#27290=LINE ( 'NONE', #5731, #19532 ) ;
#27304=CARTESIAN_POINT ( 'NONE',  ( 11.50000000000000000, 22.40709319595134730, -62.85117013414870257 ) ) ;
#27306=EDGE_CURVE ( 'NONE', #4930, #7075, #10754, .T. ) ;
#27323=ORIENTED_EDGE ( 'NONE', *, *, #3810, .T. ) ;
#27359=ORIENTED_EDGE ( 'NONE', *, *, #7073, .F. ) ;
#27438=DIRECTION ( 'NONE',  ( -1.000000000000000000, -0.000000000000000000, 0.000000000000000000 ) ) ;
#27439=CARTESIAN_POINT ( 'NONE',  ( -13.00000000000000000, 24.54213077165692525, -59.94572446259928711 ) ) ;
#27497=VECTOR ( 'NONE', #9097, 1000.000000000000114 ) ;
#27504=CIRCLE ( 'NONE', #5900, 2.000000000000000000 ) ;
#27516=CARTESIAN_POINT ( 'NONE',  ( 11.26179938798771474, 26.42151601322854759, -59.26168417594740134 ) ) ;
#27540=CARTESIAN_POINT ( 'NONE',  ( 6.585786437629999490, -16.41511111490214603, -74.85294138696069410 ) ) ;
#27566=VECTOR ( 'NONE', #724, 1000.000000000000114 ) ;
#27588=ORIENTED_EDGE ( 'NONE', *, *, #24497, .F. ) ;
#27624=ORIENTED_EDGE ( 'NONE', *, *, #3481, .F. ) ;
#27639=CARTESIAN_POINT ( 'NONE',  ( -6.771817672307487435, -16.24036849850417141, -74.78934027593398071 ) ) ;
#27678=PLANE ( 'NONE',  #29300 ) ;
#27729=PLANE ( 'NONE',  #1758 ) ;
#27743=ORIENTED_EDGE ( 'NONE', *, *, #30631, .F. ) ;
#27756=ADVANCED_FACE ( 'NONE', ( #3067 ), #4972, .T. ) ;
#27773=CARTESIAN_POINT ( 'NONE',  ( 3.607555131306940499, 0.2156355436844743512, -68.79984462960774749 ) ) ;
#27778=VECTOR ( 'NONE', #12897, 1000.000000000000114 ) ;
#27812=DIRECTION ( 'NONE',  ( 1.000000000000000000, -0.000000000000000000, 0.000000000000000000 ) ) ;
#27820=VECTOR ( 'NONE', #13372, 1000.000000000000114 ) ;
#27853=CARTESIAN_POINT ( 'NONE',  ( -3.061185584113674807, -2.905325888027505687, -69.93578169304477399 ) ) ;
#27860=ORIENTED_EDGE ( 'NONE', *, *, #14934, .F. ) ;
#27960=CARTESIAN_POINT ( 'NONE',  ( -4.000000000000000000, -29.96004123392021157, -79.78289277550334191 ) ) ;
#28014=CARTESIAN_POINT ( 'NONE',  ( 10.00000000000000000, 22.40709319595134730, -62.85117013414870257 ) ) ;
#28019=ORIENTED_EDGE ( 'NONE', *, *, #8610, .F. ) ;
#28055=ORIENTED_EDGE ( 'NONE', *, *, #25806, .T. ) ;
#28084=DIRECTION ( 'NONE',  ( 0.000000000000000000, 0.3420201433259318913, -0.9396926207858126157 ) ) ;
#28085=VERTEX_POINT ( 'NONE', #7451 ) ;
#28093=CARTESIAN_POINT ( 'NONE',  ( 2.063649162913283597, 2.140644056835441233, -68.09919883011119168 ) ) ;
#28189=EDGE_CURVE ( 'NONE', #7467, #20783, #27111, .T. ) ;
#28225=PLANE ( 'NONE',  #1248 ) ;
#28241=PRODUCT ( 'Release Lever', 'Release Lever', '', ( #639 ) ) ;
#28242=CARTESIAN_POINT ( 'NONE',  ( 3.686970300939999667, -0.1862064327014488485, -68.94610314789109395 ) ) ;
#28249=ORIENTED_EDGE ( 'NONE', *, *, #22973, .T. ) ;
#28316=LINE ( 'NONE', #23296, #6216 ) ;
#28319=CARTESIAN_POINT ( 'NONE',  ( 4.132574650175937059, -31.83942647549183746, -80.46693306215520636 ) ) ;
#28353=FACE_BOUND ( 'NONE', #22244, .T. ) ;
#28354=LINE ( 'NONE', #9000, #22348 ) ;
#28393=CYLINDRICAL_SURFACE ( 'NONE', #129, 3.749999999999999556 ) ;
#28397=DIRECTION ( 'NONE',  ( 0.000000000000000000, 0.3420201433259318358, -0.9396926207858125046 ) ) ;
#28404=EDGE_CURVE ( 'NONE', #24784, #6473, #6452, .T. ) ;
#28474=EDGE_LOOP ( 'NONE', ( #23468, #1895, #16864, #25703, #23154, #20549 ) ) ;
#28486=CARTESIAN_POINT ( 'NONE',  ( 0.000000000000000000, 26.42151601322854759, -59.26168417594741555 ) ) ;
#28509=FACE_OUTER_BOUND ( 'NONE', #15587, .T. ) ;
#28514=ADVANCED_FACE ( 'NONE', ( #25018 ), #27678, .F. ) ;
#28533=CARTESIAN_POINT ( 'NONE',  ( 0.6731456008920000400, -3.434453875705480108, -72.25672407562892374 ) ) ;
#28537=EDGE_LOOP ( 'NONE', ( #20208, #28619, #17895, #5705 ) ) ;
#28556=ORIENTED_EDGE ( 'NONE', *, *, #30368, .T. ) ;
#28619=ORIENTED_EDGE ( 'NONE', *, *, #29371, .T. ) ;
#28624=CYLINDRICAL_SURFACE ( 'NONE', #20678, 2.000000000000003553 ) ;
#28631=CARTESIAN_POINT ( 'NONE',  ( 11.00000000000000000, 27.10555629988041204, -61.14106941751904856 ) ) ;
#28663=ADVANCED_FACE ( 'NONE', ( #11252 ), #25428, .T. ) ;
#28683=CARTESIAN_POINT ( 'NONE',  ( -0.8668912886149129360, 2.622943012334922219, -67.92365636629153869 ) ) ;
#28684=EDGE_LOOP ( 'NONE', ( #16021, #11226, #23990, #6133 ) ) ;
#28705=CARTESIAN_POINT ( 'NONE',  ( 11.00000000000000000, 25.22617105830878614, -61.82510970417090590 ) ) ;
#28739=CARTESIAN_POINT ( 'NONE',  ( -6.398352591652365362, -16.59129340813300502, -74.91706649750152280 ) ) ;
#28744=PLANE ( 'NONE',  #6915 ) ;
#28760=AXIS2_PLACEMENT_3D ( 'NONE', #10490, #8735, #3706 ) ;
#28775=ORIENTED_EDGE ( 'NONE', *, *, #8409, .F. ) ;
#28776=CARTESIAN_POINT ( 'NONE',  ( 6.052054646587431641, -17.25211205318136720, -75.15758481454749074 ) ) ;
#28794=CYLINDRICAL_SURFACE ( 'NONE', #6585, 1.999999999999999334 ) ;
#28798=CARTESIAN_POINT ( 'NONE',  ( 13.00000000000000000, 23.13259184047820582, -60.45875467758818189 ) ) ;
#28827=CARTESIAN_POINT ( 'NONE',  ( -2.064060864691235508, 2.140523675421532879, -68.09924264536260807 ) ) ;
#28843=DIRECTION ( 'NONE',  ( 0.000000000000000000, -0.3420201433259318913, 0.9396926207858126157 ) ) ;
#28851=CIRCLE ( 'NONE', #8215, 2.000000000000000000 ) ;
#28902=FACE_OUTER_BOUND ( 'NONE', #17078, .T. ) ;
#28922=CARTESIAN_POINT ( 'NONE',  ( 10.00000000000000000, -13.30122639390952877, -75.84793558053411289 ) ) ;
#28969=CARTESIAN_POINT ( 'NONE',  ( 13.00000000000000000, 24.54213077165692525, -59.94572446259928711 ) ) ;
#28980=EDGE_LOOP ( 'NONE', ( #17573, #24991, #14373, #25755 ) ) ;
#28989=EDGE_CURVE ( 'NONE', #18765, #9238, #4198, .T. ) ;
#29029=DIRECTION ( 'NONE',  ( 1.000000000000000000, 0.000000000000000000, 0.000000000000000000 ) ) ;
#29048=ADVANCED_FACE ( 'NONE', ( #28353, #28509 ), #20965, .T. ) ;
#29055=VERTEX_POINT ( 'NONE', #23497 ) ;
#29083=CARTESIAN_POINT ( 'NONE',  ( 8.000000000050000892, -13.30122639390952877, -75.84793558053411289 ) ) ;
#29106=LINE ( 'NONE', #7398, #9430 ) ;
#29115=VERTEX_POINT ( 'NONE', #14972 ) ;
#29141=CARTESIAN_POINT ( 'NONE',  ( 2.664535259099999805E-15, 2.694277338339796213, -67.89769279494430521 ) ) ;
#29142=VERTEX_POINT ( 'NONE', #12598 ) ;
#29150=CARTESIAN_POINT ( 'NONE',  ( -13.00000000000000178, 24.78814172467860644, -59.85618379839584691 ) ) ;
#29152=FACE_OUTER_BOUND ( 'NONE', #21251, .T. ) ;
#29193=CARTESIAN_POINT ( 'NONE',  ( -8.000000000000000000, -15.86465192213301556, -74.65259062561435144 ) ) ;
#29203=DIRECTION ( 'NONE',  ( 1.000000000000000000, 0.000000000000000000, 0.000000000000000000 ) ) ;
#29259=EDGE_CURVE ( 'NONE', #18513, #23194, #15272, .T. ) ;
#29262=AXIS2_PLACEMENT_3D ( 'NONE', #24871, #3449, #10394 ) ;
#29286=ORIENTED_EDGE ( 'NONE', *, *, #18343, .F. ) ;
#29290=SURFACE_STYLE_FILL_AREA ( #10109 ) ;
#29299=CARTESIAN_POINT ( 'NONE',  ( -6.585786437629999490, -16.41511111490214603, -74.85294138696069410 ) ) ;
#29300=AXIS2_PLACEMENT_3D ( 'NONE', #10695, #20289, #29893 ) ;
#29314=DIRECTION ( 'NONE',  ( 0.000000000000000000, -0.3420201433259318913, 0.9396926207858126157 ) ) ;
#29326=CARTESIAN_POINT ( 'NONE',  ( -6.000000000000000000, -15.18061163548115466, -76.53197586718597734 ) ) ;
#29364=VECTOR ( 'NONE', #27812, 1000.000000000000000 ) ;
#29371=EDGE_CURVE ( 'NONE', #8103, #359, #767, .T. ) ;
#29385=EDGE_CURVE ( 'NONE', #2672, #26555, #1890, .T. ) ;
#29409=VERTEX_POINT ( 'NONE', #23613 ) ;
#29447=B_SPLINE_CURVE_WITH_KNOTS ( 'NONE', 3,
 ( #29141, #31049, #28683, #60, #28827, #7286, #3630, #22538, #5532, #22682 ),
 .UNSPECIFIED., .F., .F.,
 ( 4, 2, 2, 2, 4 ),
 ( 0.000000000000000000, 0.2500000000000000000, 0.4999999999999999445, 0.7500000000000000000, 1.000000000000000000 ),
 .UNSPECIFIED. ) ;
#29457=CYLINDRICAL_SURFACE ( 'NONE', #1496, 2.000000000000004441 ) ;
#29465=DIRECTION ( 'NONE',  ( -1.000000000000000000, 0.000000000000000000, 0.000000000000000000 ) ) ;
#29474=CARTESIAN_POINT ( 'NONE',  ( -6.000000000000000000, -17.05999687705277879, -77.21601615383784178 ) ) ;
#29490=DIRECTION ( 'NONE',  ( 0.000000000000000000, 0.3420201433259318913, -0.9396926207858126157 ) ) ;
#29497=EDGE_CURVE ( 'NONE', #3121, #18573, #2814, .T. ) ;
#29510=CARTESIAN_POINT ( 'NONE',  ( 11.00000000000000000, 25.22617105830878614, -61.82510970417090590 ) ) ;
#29525=VERTEX_POINT ( 'NONE', #4870 ) ;
#29571=AXIS2_PLACEMENT_3D ( 'NONE', #139, #4853, #26560 ) ;
#29576=CARTESIAN_POINT ( 'NONE',  ( -10.00000000000000000, -13.30122639390952877, -75.84793558053411289 ) ) ;
#29596=B_SPLINE_CURVE_WITH_KNOTS ( 'NONE', 3,
 ( #29193, #118, #7493, #16929, #5589, #15190 ),
 .UNSPECIFIED., .F., .F.,
 ( 4, 2, 4 ),
 ( 0.000000000000000000, 0.5000000000000000000, 1.000000000000000000 ),
 .UNSPECIFIED. ) ;
#29597=LINE ( 'NONE', #20001, #22870 ) ;
#29599=ORIENTED_EDGE ( 'NONE', *, *, #28189, .F. ) ;
#29613=DIRECTION ( 'NONE',  ( -0.7071067811865469066, -0.6644630243886066046, -0.2418447626481643187 ) ) ;
#29726=CARTESIAN_POINT ( 'NONE',  ( 13.00000000000000000, 24.88415091498285747, -60.88541708338509295 ) ) ;
#29763=CARTESIAN_POINT ( 'NONE',  ( -11.00000000000000000, 26.42151601322854759, -59.26168417594741555 ) ) ;
#29777=VERTEX_POINT ( 'NONE', #2167 ) ;
#29779=VECTOR ( 'NONE', #9345, 1000.000000000000114 ) ;
#29786=ORIENTED_EDGE ( 'NONE', *, *, #2695, .F. ) ;
#29789=B_SPLINE_CURVE_WITH_KNOTS ( 'NONE', 3,
 ( #1573, #27516, #15556, #25166, #25325, #6118 ),
 .UNSPECIFIED., .F., .F.,
 ( 4, 2, 4 ),
 ( 0.000000000000000000, 0.5000000000000000000, 1.000000000000000000 ),
 .UNSPECIFIED. ) ;
#29804=ORIENTED_EDGE ( 'NONE', *, *, #16999, .T. ) ;
#29850=CARTESIAN_POINT ( 'NONE',  ( 0.000000000000000000, 27.10555629988041204, -61.14106941751904856 ) ) ;
#29890=EDGE_CURVE ( 'NONE', #5989, #13375, #12730, .T. ) ;
#29893=DIRECTION ( 'NONE',  ( 0.000000000000000000, -0.3420201433259318358, 0.9396926207858125046 ) ) ;
#29901=ORIENTED_EDGE ( 'NONE', *, *, #21022, .F. ) ;
#29905=CARTESIAN_POINT ( 'NONE',  ( -4.520688084463085232, -31.79175087150127510, -80.44958056140195879 ) ) ;
#29936=ORIENTED_EDGE ( 'NONE', *, *, #3201, .T. ) ;
#29962=LINE ( 'NONE', #17677, #27566 ) ;
#29963=ORIENTED_EDGE ( 'NONE', *, *, #4587, .F. ) ;
#29964=CYLINDRICAL_SURFACE ( 'NONE', #27245, 3.749999999999999556 ) ;
#29987=ORIENTED_EDGE ( 'NONE', *, *, #16182, .F. ) ;
#30002=PLANE ( 'NONE',  #13500 ) ;
#30114=FACE_BOUND ( 'NONE', #28474, .T. ) ;
#30129=CARTESIAN_POINT ( 'NONE',  ( 8.000000000000000000, -17.74403716370463968, -75.33663091226621589 ) ) ;
#30156=CARTESIAN_POINT ( 'NONE',  ( 7.476504230907038639, -15.91356728955108046, -74.67039436335275582 ) ) ;
#30165=CARTESIAN_POINT ( 'NONE',  ( 0.000000000000000000, 4.811145170119999648, -67.12721591429999535 ) ) ;
#30295=EDGE_LOOP ( 'NONE', ( #168, #28556, #23691, #14580 ) ) ;
#30323=CARTESIAN_POINT ( 'NONE',  ( 9.414213562409999625, -15.31419272936388687, -74.45223986426802298 ) ) ;
#30355=EDGE_CURVE ( 'NONE', #25829, #26031, #17476, .T. ) ;
#30368=EDGE_CURVE ( 'NONE', #21919, #10856, #1710, .T. ) ;
#30409=FACE_OUTER_BOUND ( 'NONE', #24383, .T. ) ;
#30432=EDGE_LOOP ( 'NONE', ( #20508, #12828, #29987, #12723 ) ) ;
#30452=DIRECTION ( 'NONE',  ( 0.000000000000000000, -0.3420201433259318913, 0.9396926207858126157 ) ) ;
#30465=B_SPLINE_CURVE_WITH_KNOTS ( 'NONE', 3,
 ( #430, #116, #17084, #4976, #7638, #9695, #22276, #17235 ),
 .UNSPECIFIED., .F., .F.,
 ( 4, 2, 2, 4 ),
 ( 0.000000000000000000, 0.2500000000000001665, 0.5000000000000003331, 1.000000000000000000 ),
 .UNSPECIFIED. ) ;
#30524=LINE ( 'NONE', #3924, #2942 ) ;
#30560=ORIENTED_EDGE ( 'NONE', *, *, #7464, .T. ) ;
#30599=ORIENTED_EDGE ( 'NONE', *, *, #27, .F. ) ;
#30611=CARTESIAN_POINT ( 'NONE',  ( 7.000000000000000000, -15.86465192213301556, -74.65259062561435144 ) ) ;
#30622=EDGE_CURVE ( 'NONE', #9238, #27093, #1791, .T. ) ;
#30623=CARTESIAN_POINT ( 'NONE',  ( 0.2188333036866983439, 2.694277338339796657, -67.89769279494433363 ) ) ;
#30631=EDGE_CURVE ( 'NONE', #16796, #14059, #25709, .T. ) ;
#30637=LINE ( 'NONE', #15844, #9472 ) ;
#30663=ORIENTED_EDGE ( 'NONE', *, *, #9957, .F. ) ;
#30670=AXIS2_PLACEMENT_3D ( 'NONE', #13856, #6767, #16363 ) ;
#30722=DIRECTION ( 'NONE',  ( -1.000000000000000000, 0.000000000000000000, 0.000000000000000000 ) ) ;
#30745=ORIENTED_EDGE ( 'NONE', *, *, #7073, .T. ) ;
#30746=ADVANCED_FACE ( 'NONE', ( #16703 ), #14370, .F. ) ;
#30764=PLANE ( 'NONE',  #23677 ) ;
#30767=PRODUCT_DEFINITION_SHAPE ( 'NONE', 'NONE',  #24622 ) ;
#30787=CARTESIAN_POINT ( 'NONE',  ( 6.000000000000000000, -29.96004123392021157, -79.78289277550334191 ) ) ;
#30801=EDGE_CURVE ( 'NONE', #29409, #23194, #17791, .T. ) ;
#30806=DIRECTION ( 'NONE',  ( 0.000000000000000000, -0.9396926207858125046, -0.3420201433259318358 ) ) ;
#30920=DIRECTION ( 'NONE',  ( 0.000000000000000000, -0.3420201433259318913, 0.9396926207858126157 ) ) ;
#30931=LINE ( 'NONE', #26205, #5451 ) ;
#30999=CARTESIAN_POINT ( 'NONE',  ( -2.220446049249999755E-16, -0.1455297029551360921, -71.05965357398815740 ) ) ;
#31015=FACE_OUTER_BOUND ( 'NONE', #28537, .T. ) ;
#31028=AXIS2_PLACEMENT_3D ( 'NONE', #23751, #24359, #19329 ) ;
#31049=CARTESIAN_POINT ( 'NONE',  ( -0.4334975989126229612, 2.694277338339795769, -67.89769279494433363 ) ) ;
#31074=DIRECTION ( 'NONE',  ( 0.000000000000000000, 0.3420201433259318358, -0.9396926207858125046 ) ) ;
#31083=ORIENTED_EDGE ( 'NONE', *, *, #30622, .T. ) ;
#31086=VERTEX_POINT ( 'NONE', #13380 ) ;
#31098=ORIENTED_EDGE ( 'NONE', *, *, #23903, .T. ) ;
#31113=CARTESIAN_POINT ( 'NONE',  ( -4.000000000000000000, -29.96004123392021157, -79.78289277550334191 ) ) ;
ENDSEC;
END-ISO-10303-21;
